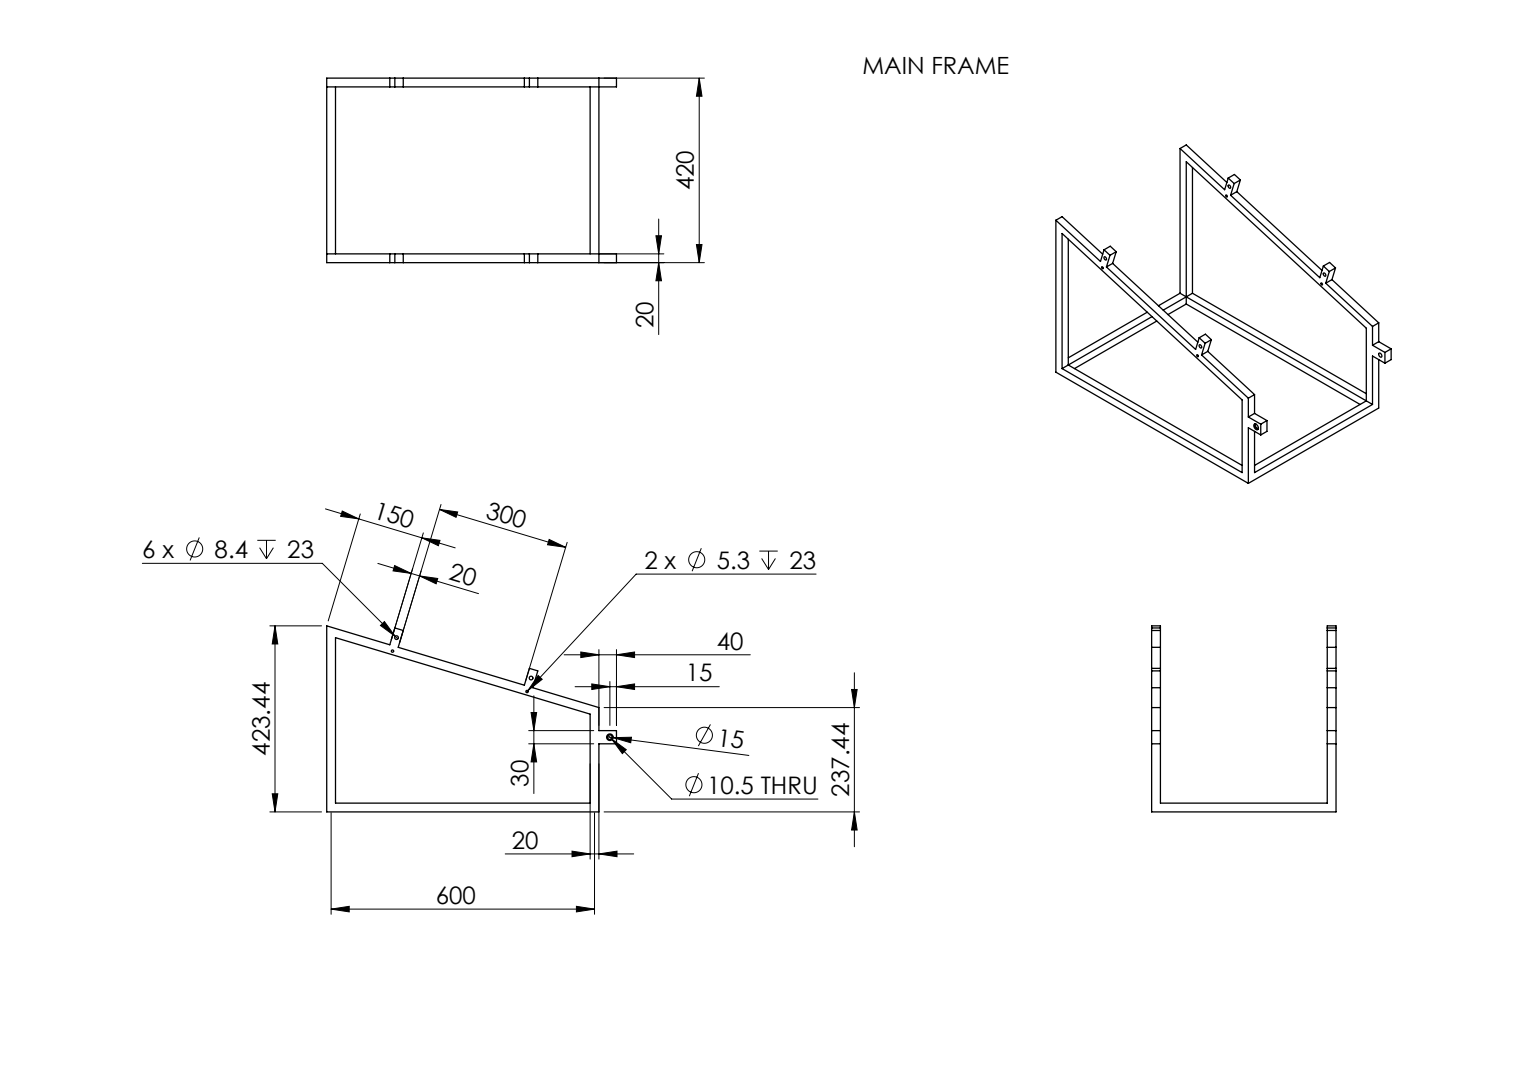
ISO-10303-21;
HEADER;
FILE_DESCRIPTION (('STEP AP214'),
    '1' );
FILE_NAME ('main frame.step',
    '2026-10-27T17:01:19',
    ( '' ),
    ( '' ),
    'SwSTEP 2.0',
    'SolidWorks 2026',
    '' );
FILE_SCHEMA (( 'AUTOMOTIVE_DESIGN' ));
ENDSEC;

DATA;
#2=DIRECTION ( 'NONE',  ( 1.000000000000000000, 0.000000000000000000, 0.000000000000000000 ) ) ;
#7=EDGE_CURVE ( 'NONE', #11993, #2660, #12348, .T. ) ;
#12=ORIENTED_EDGE ( 'NONE', *, *, #9612, .F. ) ;
#21=CARTESIAN_POINT ( 'NONE',  ( 148.9991633467111569, 386.6211705227183870, -190.0000000000000000 ) ) ;
#26=DIRECTION ( 'NONE',  ( 0.000000000000000000, 0.000000000000000000, 1.000000000000000000 ) ) ;
#34=EDGE_CURVE ( 'NONE', #1936, #10044, #4903, .T. ) ;
#41=CARTESIAN_POINT ( 'NONE',  ( 164.3243839102495656, 402.9042173714779551, -210.0000000000000000 ) ) ;
#50=EDGE_LOOP ( 'NONE', ( #5774, #9979, #12011, #287 ) ) ;
#54=VERTEX_POINT ( 'NONE', #6074 ) ;
#72=VERTEX_POINT ( 'NONE', #2614 ) ;
#74=EDGE_LOOP ( 'NONE', ( #5773, #12707 ) ) ;
#76=CARTESIAN_POINT ( 'NONE',  ( 451.6722694765949768, 316.6998517015743460, -210.0000000000000000 ) ) ;
#79=CARTESIAN_POINT ( 'NONE',  ( 650.0000000000000000, 175.0000000000000568, 190.0000000000000000 ) ) ;
#80=CARTESIAN_POINT ( 'NONE',  ( 459.7035746174795463, 294.6698471414878782, 210.0000000000000000 ) ) ;
#82=DIRECTION ( 'NONE',  ( 1.000000000000000000, 0.000000000000000000, 0.000000000000000000 ) ) ;
#84=ORIENTED_EDGE ( 'NONE', *, *, #4575, .F. ) ;
#85=CARTESIAN_POINT ( 'NONE',  ( 642.5000000000001137, 160.0000000000000284, -207.0000000000000000 ) ) ;
#90=DIRECTION ( 'NONE',  ( 1.000000000000000000, 0.000000000000000000, 0.000000000000000000 ) ) ;
#103=CARTESIAN_POINT ( 'NONE',  ( 642.4999005938085475, 159.0059381730093548, -210.0000000000000284 ) ) ;
#104=CARTESIAN_POINT ( 'NONE',  ( 642.5000000000001137, 160.0000000000000284, 210.0000119999999981 ) ) ;
#105=LINE ( 'NONE', #11206, #8037 ) ;
#116=CARTESIAN_POINT ( 'NONE',  ( 145.1678582058265476, 408.6511750828048548, -190.0000000000000000 ) ) ;
#130=EDGE_CURVE ( 'NONE', #2847, #2989, #365, .T. ) ;
#132=CARTESIAN_POINT ( 'NONE',  ( 610.0000000000000000, 0.000000000000000000, -210.0000000000000000 ) ) ;
#134=CARTESIAN_POINT ( 'NONE',  ( 650.0000000000000000, 0.000000000000000000, 0.000000000000000000 ) ) ;
#137=CARTESIAN_POINT ( 'NONE',  ( 641.5533979126569193, 156.2228576472182624, 210.0000119999999981 ) ) ;
#140=CARTESIAN_POINT ( 'NONE',  ( 9.498873539028489220E-16, -10.00000000000000000, 210.0000000000000000 ) ) ;
#144=VECTOR ( 'NONE', #10565, 1000.000000000000000 ) ;
#145=VERTEX_POINT ( 'NONE', #14118 ) ;
#153=EDGE_LOOP ( 'NONE', ( #10187, #6954 ) ) ;
#165=CARTESIAN_POINT ( 'NONE',  ( 459.3348797583642522, 272.6398425814014104, -210.0000000000000000 ) ) ;
#176=VECTOR ( 'NONE', #3313, 1000.000000000000000 ) ;
#180=ORIENTED_EDGE ( 'NONE', *, *, #12151, .F. ) ;
#187=ORIENTED_EDGE ( 'NONE', *, *, #791, .F. ) ;
#197=VERTEX_POINT ( 'NONE', #7549 ) ;
#202=VECTOR ( 'NONE', #5695, 1000.000000000000000 ) ;
#205=LINE ( 'NONE', #12625, #7486 ) ;
#210=DIRECTION ( 'NONE',  ( 0.000000000000000000, 0.000000000000000000, 1.000000000000000000 ) ) ;
#213=DIRECTION ( 'NONE',  ( 0.000000000000000000, -0.000000000000000000, -1.000000000000000000 ) ) ;
#214=VERTEX_POINT ( 'NONE', #14200 ) ;
#216=CARTESIAN_POINT ( 'NONE',  ( 640.9975013179864618, 155.3908996001881064, 210.0000119999999981 ) ) ;
#217=CARTESIAN_POINT ( 'NONE',  ( 145.1678582058265192, 408.6511750828049117, 210.0000000000000000 ) ) ;
#235=AXIS2_PLACEMENT_3D ( 'NONE', #506, #13872, #10410 ) ;
#236=DIRECTION ( 'NONE',  ( 0.000000000000000000, 0.000000000000000000, 1.000000000000000000 ) ) ;
#244=DIRECTION ( 'NONE',  ( 0.9578262852211513190, -0.2873478855663453846, 0.000000000000000000 ) ) ;
#254=CARTESIAN_POINT ( 'NONE',  ( 10.00000000000000000, 0.000000000000000000, 210.0000000000000000 ) ) ;
#257=ORIENTED_EDGE ( 'NONE', *, *, #4905, .T. ) ;
#258=CARTESIAN_POINT ( 'NONE',  ( 10.00000000000000000, 386.5596934910894902, -190.0000000000000000 ) ) ;
#261=LINE ( 'NONE', #1530, #10839 ) ;
#262=DIRECTION ( 'NONE',  ( -0.000000000000000000, -0.000000000000000000, -1.000000000000000000 ) ) ;
#263=VECTOR ( 'NONE', #2526, 1000.000000000000000 ) ;
#265=CARTESIAN_POINT ( 'NONE',  ( 459.7035746174795463, 294.6698471414878782, -210.0000000000000000 ) ) ;
#281=EDGE_CURVE ( 'NONE', #5961, #525, #3049, .T. ) ;
#283=CARTESIAN_POINT ( 'NONE',  ( 112.9652219749295341, 376.5507399164317803, -190.0000000000000000 ) ) ;
#285=VECTOR ( 'NONE', #13609, 1000.000000000000000 ) ;
#287=ORIENTED_EDGE ( 'NONE', *, *, #8174, .T. ) ;
#291=LINE ( 'NONE', #8346, #11794 ) ;
#292=ORIENTED_EDGE ( 'NONE', *, *, #6303, .T. ) ;
#300=CARTESIAN_POINT ( 'NONE',  ( 650.0000000000000000, 175.0000000000000568, 210.0000000000000000 ) ) ;
#311=EDGE_CURVE ( 'NONE', #1794, #10356, #7010, .T. ) ;
#313=LINE ( 'NONE', #2471, #1913 ) ;
#320=CARTESIAN_POINT ( 'NONE',  ( 440.1783540539412343, 278.3868002927283101, -190.0000000000000000 ) ) ;
#322=EDGE_CURVE ( 'NONE', #11174, #11494, #10043, .T. ) ;
#324=VECTOR ( 'NONE', #11210, 1000.000000000000000 ) ;
#326=ORIENTED_EDGE ( 'NONE', *, *, #6236, .F. ) ;
#336=CARTESIAN_POINT ( 'NONE',  ( 145.1678582058265192, 408.6511750828049117, 210.0000000000000000 ) ) ;
#337=ORIENTED_EDGE ( 'NONE', *, *, #5739, .T. ) ;
#338=FACE_OUTER_BOUND ( 'NONE', #7888, .T. ) ;
#343=ORIENTED_EDGE ( 'NONE', *, *, #2161, .T. ) ;
#347=EDGE_CURVE ( 'NONE', #8605, #12947, #205, .T. ) ;
#352=VERTEX_POINT ( 'NONE', #14549 ) ;
#359=EDGE_LOOP ( 'NONE', ( #3831, #5633, #326, #12007 ) ) ;
#363=ORIENTED_EDGE ( 'NONE', *, *, #918, .F. ) ;
#365=LINE ( 'NONE', #2825, #10917 ) ;
#384=FACE_OUTER_BOUND ( 'NONE', #5110, .T. ) ;
#385=ORIENTED_EDGE ( 'NONE', *, *, #3968, .F. ) ;
#386=CARTESIAN_POINT ( 'NONE',  ( 10.00000000000000000, 386.5596934910894902, 210.0000000000000000 ) ) ;
#387=LINE ( 'NONE', #4789, #930 ) ;
#393=ORIENTED_EDGE ( 'NONE', *, *, #10167, .F. ) ;
#396=ORIENTED_EDGE ( 'NONE', *, *, #10216, .T. ) ;
#397=EDGE_CURVE ( 'NONE', #6493, #1729, #8054, .T. ) ;
#398=CIRCLE ( 'NONE', #12374, 4.200000000000009059 ) ;
#413=DIRECTION ( 'NONE',  ( -0.9578262852211513190, 0.2873478855663453846, 0.000000000000000000 ) ) ;
#414=ORIENTED_EDGE ( 'NONE', *, *, #14037, .F. ) ;
#417=ORIENTED_EDGE ( 'NONE', *, *, #9564, .F. ) ;
#432=AXIS2_PLACEMENT_3D ( 'NONE', #1047, #4454, #8952 ) ;
#437=CARTESIAN_POINT ( 'NONE',  ( 610.0000000000000000, 10.00000000000005507, -190.0000000000000000 ) ) ;
#441=CARTESIAN_POINT ( 'NONE',  ( 650.0000000000000000, 175.0000000000000568, -210.0000000000000000 ) ) ;
#444=CARTESIAN_POINT ( 'NONE',  ( 642.3047950750122936, 158.0368908673054023, 210.0000119999999981 ) ) ;
#459=LINE ( 'NONE', #6230, #3858 ) ;
#463=DIRECTION ( 'NONE',  ( 0.000000000000000000, 0.000000000000000000, -1.000000000000000000 ) ) ;
#466=AXIS2_PLACEMENT_3D ( 'NONE', #4153, #9690, #6360 ) ;
#472=EDGE_CURVE ( 'NONE', #11723, #11023, #398, .T. ) ;
#473=CARTESIAN_POINT ( 'NONE',  ( 459.7035746174796031, 294.6698471414878782, 210.0000000000000000 ) ) ;
#476=ORIENTED_EDGE ( 'NONE', *, *, #1979, .F. ) ;
#480=DIRECTION ( 'NONE',  ( -0.000000000000000000, -0.000000000000000000, -1.000000000000000000 ) ) ;
#484=VECTOR ( 'NONE', #9358, 1000.000000000000000 ) ;
#489=VECTOR ( 'NONE', #7910, 1000.000000000000114 ) ;
#493=EDGE_CURVE ( 'NONE', #6798, #4861, #9598, .T. ) ;
#498=EDGE_CURVE ( 'NONE', #10448, #9080, #1487, .T. ) ;
#499=CARTESIAN_POINT ( 'NONE',  ( 635.0000000000000000, 160.0000000000000284, -210.0000000000000000 ) ) ;
#503=VERTEX_POINT ( 'NONE', #14036 ) ;
#506=CARTESIAN_POINT ( 'NONE',  ( 455.5035746174796714, 294.6698471414878782, -210.0000000000000000 ) ) ;
#517=EDGE_LOOP ( 'NONE', ( #8251, #6381, #5116, #1964 ) ) ;
#525=VERTEX_POINT ( 'NONE', #9313 ) ;
#528=DIRECTION ( 'NONE',  ( -1.000000000000000000, 0.000000000000000000, 0.000000000000000000 ) ) ;
#529=VECTOR ( 'NONE', #13044, 1000.000000000000000 ) ;
#534=CYLINDRICAL_SURFACE ( 'NONE', #9490, 4.199999999999926459 ) ;
#536=CARTESIAN_POINT ( 'NONE',  ( 650.0000000000000000, 145.0000000000000568, -210.0000000000000000 ) ) ;
#542=VERTEX_POINT ( 'NONE', #1550 ) ;
#550=DIRECTION ( 'NONE',  ( 0.9578262852211513190, -0.2873478855663453846, 0.000000000000000000 ) ) ;
#562=FACE_BOUND ( 'NONE', #4810, .T. ) ;
#565=ORIENTED_EDGE ( 'NONE', *, *, #4113, .T. ) ;
#577=CARTESIAN_POINT ( 'NONE',  ( 590.0000000000000000, -9.999999999999941380, -190.0000000000000000 ) ) ;
#586=ORIENTED_EDGE ( 'NONE', *, *, #12930, .F. ) ;
#589=CARTESIAN_POINT ( 'NONE',  ( 610.0000000000000000, 0.000000000000000000, 210.0000000000000000 ) ) ;
#594=ADVANCED_FACE ( 'NONE', ( #8569 ), #6567, .F. ) ;
#606=CARTESIAN_POINT ( 'NONE',  ( 451.3035746174797396, 294.6698471414878782, 210.0000000000000000 ) ) ;
#608=DIRECTION ( 'NONE',  ( 0.000000000000000000, 0.000000000000000000, -1.000000000000000000 ) ) ;
#613=CARTESIAN_POINT ( 'NONE',  ( 639.6091003998118367, 165.9975013179864334, 210.0000119999999981 ) ) ;
#619=PLANE ( 'NONE',  #5173 ) ;
#620=ORIENTED_EDGE ( 'NONE', *, *, #10389, .T. ) ;
#624=DIRECTION ( 'NONE',  ( -0.000000000000000000, -0.000000000000000000, -1.000000000000000000 ) ) ;
#634=( NAMED_UNIT ( * ) SI_UNIT ( $, .STERADIAN. ) SOLID_ANGLE_UNIT ( ) );
#646=CARTESIAN_POINT ( 'NONE',  ( 639.6004632909515522, 166.0062790084377013, -210.0000000000000000 ) ) ;
#650=ORIENTED_EDGE ( 'NONE', *, *, #6792, .F. ) ;
#656=CARTESIAN_POINT ( 'NONE',  ( 112.9652219749295341, 376.5507399164317803, 210.0000000000000000 ) ) ;
#657=ORIENTED_EDGE ( 'NONE', *, *, #4005, .F. ) ;
#674=PLANE ( 'NONE',  #14348 ) ;
#675=EDGE_LOOP ( 'NONE', ( #11557, #8430, #2756, #7355 ) ) ;
#685=DIRECTION ( 'NONE',  ( 0.000000000000000000, 1.000000000000000000, 0.000000000000000000 ) ) ;
#691=CARTESIAN_POINT ( 'NONE',  ( 631.2228576472183477, 166.5533979126570330, 210.0000119999999981 ) ) ;
#703=CIRCLE ( 'NONE', #8021, 4.199999999999981526 ) ;
#713=CARTESIAN_POINT ( 'NONE',  ( 142.4540310085880606, 355.9707293956415697, -210.0000000000000000 ) ) ;
#722=ORIENTED_EDGE ( 'NONE', *, *, #12878, .F. ) ;
#725=DIRECTION ( 'NONE',  ( -1.000000000000000000, 0.000000000000000000, 0.000000000000000000 ) ) ;
#735=DIRECTION ( 'NONE',  ( 1.000000000000000000, 0.000000000000000000, 0.000000000000000000 ) ) ;
#739=VERTEX_POINT ( 'NONE', #10988 ) ;
#750=ORIENTED_EDGE ( 'NONE', *, *, #10896, .T. ) ;
#757=CARTESIAN_POINT ( 'NONE',  ( 640.2500000000000000, 160.0000000000000284, -190.0000000000000000 ) ) ;
#770=ORIENTED_EDGE ( 'NONE', *, *, #10512, .T. ) ;
#776=VECTOR ( 'NONE', #6967, 1000.000000000000000 ) ;
#779=CYLINDRICAL_SURFACE ( 'NONE', #2321, 7.500000000000062172 ) ;
#780=ORIENTED_EDGE ( 'NONE', *, *, #4466, .T. ) ;
#781=FACE_OUTER_BOUND ( 'NONE', #3795, .T. ) ;
#791=EDGE_CURVE ( 'NONE', #6358, #5212, #2203, .T. ) ;
#793=VERTEX_POINT ( 'NONE', #5751 ) ;
#799=DIRECTION ( 'NONE',  ( -1.000000000000000000, 0.000000000000000000, 0.000000000000000000 ) ) ;
#800=CARTESIAN_POINT ( 'NONE',  ( 446.3084422793565409, 264.0194060144110608, -210.0000000000000000 ) ) ;
#804=CARTESIAN_POINT ( 'NONE',  ( 451.6722694765949768, 316.6998517015743460, -190.0000000000000000 ) ) ;
#813=PLANE ( 'NONE',  #12711 ) ;
#819=ADVANCED_FACE ( 'NONE', ( #11141 ), #13509, .T. ) ;
#830=ORIENTED_EDGE ( 'NONE', *, *, #10724, .T. ) ;
#842=ORIENTED_EDGE ( 'NONE', *, *, #9433, .T. ) ;
#848=LINE ( 'NONE', #5367, #4476 ) ;
#850=CARTESIAN_POINT ( 'NONE',  ( 627.5000000000000000, 160.0000000000000284, -210.0000119999999981 ) ) ;
#851=( LENGTH_UNIT ( ) NAMED_UNIT ( * ) SI_UNIT ( .MILLI., .METRE. ) );
#854=LINE ( 'NONE', #14242, #1628 ) ;
#857=ORIENTED_EDGE ( 'NONE', *, *, #6432, .F. ) ;
#871=ADVANCED_FACE ( 'NONE', ( #11787 ), #7070, .F. ) ;
#881=FACE_OUTER_BOUND ( 'NONE', #6176, .T. ) ;
#885=VECTOR ( 'NONE', #12868, 1000.000000000000000 ) ;
#902=VERTEX_POINT ( 'NONE', #5973 ) ;
#915=LINE ( 'NONE', #5298, #3326 ) ;
#918=EDGE_CURVE ( 'NONE', #12905, #9301, #11493, .T. ) ;
#919=VECTOR ( 'NONE', #3316, 1000.000000000000000 ) ;
#922=DIRECTION ( 'NONE',  ( -0.2873478855663453846, -0.9578262852211513190, -0.000000000000000000 ) ) ;
#928=ORIENTED_EDGE ( 'NONE', *, *, #12930, .T. ) ;
#929=AXIS2_PLACEMENT_3D ( 'NONE', #5591, #6707, #6495 ) ;
#930=VECTOR ( 'NONE', #8229, 1000.000000000000000 ) ;
#932=ORIENTED_EDGE ( 'NONE', *, *, #311, .T. ) ;
#937=CARTESIAN_POINT ( 'NONE',  ( 153.1991633467111456, 386.6211705227183870, 210.0000000000000000 ) ) ;
#938=CARTESIAN_POINT ( 'NONE',  ( 628.9937209914679670, 164.6004632908573342, -210.0000000000000000 ) ) ;
#947=VECTOR ( 'NONE', #14401, 1000.000000000000227 ) ;
#959=CARTESIAN_POINT ( 'NONE',  ( 590.0000000000000000, 10.00000000000005507, 210.0000000000000000 ) ) ;
#970=EDGE_CURVE ( 'NONE', #9080, #2989, #1606, .T. ) ;
#974=LINE ( 'NONE', #12475, #9641 ) ;
#976=CIRCLE ( 'NONE', #8526, 2.649999999999985700 ) ;
#980=DIRECTION ( 'NONE',  ( 0.000000000000000000, -1.000000000000000000, 0.000000000000000000 ) ) ;
#988=AXIS2_PLACEMENT_3D ( 'NONE', #13184, #5359, #12203 ) ;
#990=FACE_OUTER_BOUND ( 'NONE', #11899, .T. ) ;
#994=ORIENTED_EDGE ( 'NONE', *, *, #11063, .T. ) ;
#996=CARTESIAN_POINT ( 'NONE',  ( 10.00000000000000000, -10.00000000000000000, 190.0000000000000000 ) ) ;
#1000=EDGE_CURVE ( 'NONE', #10070, #5539, #3911, .T. ) ;
#1003=CYLINDRICAL_SURFACE ( 'NONE', #11112, 7.500000000000062172 ) ;
#1009=DIRECTION ( 'NONE',  ( 1.000000000000000000, 0.000000000000000000, -0.000000000000000000 ) ) ;
#1017=CARTESIAN_POINT ( 'NONE',  ( 627.5000000000000000, 160.9948216655610622, -210.0000000000000284 ) ) ;
#1025=LINE ( 'NONE', #1991, #8652 ) ;
#1027=FACE_OUTER_BOUND ( 'NONE', #1102, .T. ) ;
#1031=ORIENTED_EDGE ( 'NONE', *, *, #1242, .F. ) ;
#1037=EDGE_LOOP ( 'NONE', ( #8781, #13398, #8659, #1616 ) ) ;
#1038=CARTESIAN_POINT ( 'NONE',  ( 443.6584422793565636, 264.0194060144110608, -190.0000000000000000 ) ) ;
#1047=CARTESIAN_POINT ( 'NONE',  ( 455.5035746174796714, 294.6698471414878782, -190.0000000000000000 ) ) ;
#1054=DIRECTION ( 'NONE',  ( -0.000000000000000000, -0.000000000000000000, 1.000000000000000000 ) ) ;
#1055=DIRECTION ( 'NONE',  ( -0.9578262852211517631, 0.2873478855663438858, 0.000000000000000000 ) ) ;
#1062=ORIENTED_EDGE ( 'NONE', *, *, #347, .F. ) ;
#1064=CARTESIAN_POINT ( 'NONE',  ( 451.6722694765949768, 316.6998517015743460, -210.0000000000000000 ) ) ;
#1066=ADVANCED_FACE ( 'NONE', ( #9586 ), #6607, .T. ) ;
#1073=CARTESIAN_POINT ( 'NONE',  ( -10.00000000000000000, 0.000000000000000000, -190.0000000000000000 ) ) ;
#1076=( LENGTH_UNIT ( ) NAMED_UNIT ( * ) SI_UNIT ( .MILLI., .METRE. ) );
#1084=FACE_OUTER_BOUND ( 'NONE', #6931, .T. ) ;
#1085=CARTESIAN_POINT ( 'NONE',  ( 630.3996772907336208, 166.0061384269410212, -210.0000000000000284 ) ) ;
#1102=EDGE_LOOP ( 'NONE', ( #5350, #8471, #4315, #12302 ) ) ;
#1104=ORIENTED_EDGE ( 'NONE', *, *, #7956, .T. ) ;
#1111=ORIENTED_EDGE ( 'NONE', *, *, #1647, .T. ) ;
#1123=CARTESIAN_POINT ( 'NONE',  ( 10.00000000000000000, 386.5596934910894902, 210.0000000000000000 ) ) ;
#1124=EDGE_CURVE ( 'NONE', #10210, #9473, #7995, .T. ) ;
#1126=LINE ( 'NONE', #5639, #9616 ) ;
#1129=ORIENTED_EDGE ( 'NONE', *, *, #11458, .T. ) ;
#1138=VERTEX_POINT ( 'NONE', #12577 ) ;
#1145=CARTESIAN_POINT ( 'NONE',  ( 635.0000000000000000, 160.0000000000000284, 190.0000000000000284 ) ) ;
#1146=EDGE_CURVE ( 'NONE', #503, #13396, #5852, .T. ) ;
#1149=ORIENTED_EDGE ( 'NONE', *, *, #11070, .T. ) ;
#1152=CARTESIAN_POINT ( 'NONE',  ( 459.3348797583643091, 272.6398425814014104, -190.0000000000000000 ) ) ;
#1156=CIRCLE ( 'NONE', #13898, 4.199999999999981526 ) ;
#1158=DIRECTION ( 'NONE',  ( -0.000000000000000000, -0.000000000000000000, -1.000000000000000000 ) ) ;
#1181=LINE ( 'NONE', #959, #202 ) ;
#1182=CIRCLE ( 'NONE', #4025, 2.649999999999985700 ) ;
#1183=CARTESIAN_POINT ( 'NONE',  ( 650.0000000000000000, 145.0000000000000568, -190.0000000000000000 ) ) ;
#1185=CARTESIAN_POINT ( 'NONE',  ( 451.6722694765949768, 316.6998517015743460, 190.0000000000000000 ) ) ;
#1189=DIRECTION ( 'NONE',  ( 0.000000000000000000, 1.000000000000000000, 0.000000000000000000 ) ) ;
#1194=EDGE_LOOP ( 'NONE', ( #13478, #6976 ) ) ;
#1195=ORIENTED_EDGE ( 'NONE', *, *, #13922, .T. ) ;
#1198=VECTOR ( 'NONE', #12811, 1000.000000000000114 ) ;
#1205=ORIENTED_EDGE ( 'NONE', *, *, #4135, .F. ) ;
#1208=CIRCLE ( 'NONE', #13243, 7.500000000000062172 ) ;
#1211=CARTESIAN_POINT ( 'NONE',  ( 148.9991633467111569, 386.6211705227183870, 210.0000000000000000 ) ) ;
#1227=DIRECTION ( 'NONE',  ( -0.2873478855663453846, -0.9578262852211513190, -0.000000000000000000 ) ) ;
#1229=EDGE_LOOP ( 'NONE', ( #830, #13146 ) ) ;
#1242=EDGE_CURVE ( 'NONE', #72, #3152, #10578, .T. ) ;
#1244=CARTESIAN_POINT ( 'NONE',  ( 638.7885571598276329, 153.4512226587835642, -210.0000000000000000 ) ) ;
#1246=DIRECTION ( 'NONE',  ( 1.000000000000000000, 0.000000000000000000, 0.000000000000000000 ) ) ;
#1249=CARTESIAN_POINT ( 'NONE',  ( 112.9652219749295341, 376.5507399164317803, 210.0000000000000000 ) ) ;
#1251=DIRECTION ( 'NONE',  ( -0.9578262852211513190, 0.2873478855663453846, 0.000000000000000000 ) ) ;
#1260=VECTOR ( 'NONE', #3658, 1000.000000000000000 ) ;
#1262=ORIENTED_EDGE ( 'NONE', *, *, #8034, .T. ) ;
#1265=FACE_OUTER_BOUND ( 'NONE', #4449, .T. ) ;
#1267=LINE ( 'NONE', #577, #4034 ) ;
#1272=DIRECTION ( 'NONE',  ( 1.387778780781446464E-15, -2.775557561562892929E-15, 1.000000000000000000 ) ) ;
#1277=CARTESIAN_POINT ( 'NONE',  ( 630.3908996001882770, 154.0024986820136803, 210.0000119999999981 ) ) ;
#1289=ORIENTED_EDGE ( 'NONE', *, *, #8696, .F. ) ;
#1290=DIRECTION ( 'NONE',  ( -0.000000000000000000, -0.000000000000000000, 1.000000000000000000 ) ) ;
#1294=DIRECTION ( 'NONE',  ( -1.000000000000000000, -9.498873539028489960E-17, -0.000000000000000000 ) ) ;
#1297=PLANE ( 'NONE',  #3818 ) ;
#1299=PLANE ( 'NONE',  #13009 ) ;
#1306=FACE_OUTER_BOUND ( 'NONE', #4104, .T. ) ;
#1308=ORIENTED_EDGE ( 'NONE', *, *, #9612, .T. ) ;
#1313=DIRECTION ( 'NONE',  ( 0.000000000000000000, 0.000000000000000000, 1.000000000000000000 ) ) ;
#1319=VERTEX_POINT ( 'NONE', #10502 ) ;
#1326=EDGE_CURVE ( 'NONE', #12898, #12523, #9621, .T. ) ;
#1335=EDGE_CURVE ( 'NONE', #8820, #739, #4018, .T. ) ;
#1342=ORIENTED_EDGE ( 'NONE', *, *, #9115, .F. ) ;
#1356=PLANE ( 'NONE',  #5436 ) ;
#1358=EDGE_LOOP ( 'NONE', ( #5343, #14402, #10147, #3262 ) ) ;
#1378=VECTOR ( 'NONE', #1272, 1000.000000000000000 ) ;
#1379=CARTESIAN_POINT ( 'NONE',  ( 642.3095993250867650, 158.0482295922596450, -210.0000000000000000 ) ) ;
#1385=CARTESIAN_POINT ( 'NONE',  ( 459.3348797583642522, 272.6398425814014104, -210.0000000000000000 ) ) ;
#1394=ORIENTED_EDGE ( 'NONE', *, *, #5211, .F. ) ;
#1398=ORIENTED_EDGE ( 'NONE', *, *, #3960, .T. ) ;
#1402=DIRECTION ( 'NONE',  ( -0.000000000000000000, -0.000000000000000000, -1.000000000000000000 ) ) ;
#1407=DIRECTION ( 'NONE',  ( -0.000000000000000000, -0.000000000000000000, 1.000000000000000000 ) ) ;
#1414=VECTOR ( 'NONE', #13789, 1000.000000000000114 ) ;
#1416=AXIS2_PLACEMENT_3D ( 'NONE', #12274, #4328, #9037 ) ;
#1425=EDGE_CURVE ( 'NONE', #10194, #525, #4233, .T. ) ;
#1428=EDGE_CURVE ( 'NONE', #12947, #2635, #10045, .T. ) ;
#1437=AXIS2_PLACEMENT_3D ( 'NONE', #800, #13135, #14530 ) ;
#1438=ORIENTED_EDGE ( 'NONE', *, *, #12056, .T. ) ;
#1444=VECTOR ( 'NONE', #262, 1000.000000000000000 ) ;
#1447=AXIS2_PLACEMENT_3D ( 'NONE', #13346, #3239, #1833 ) ;
#1451=DIRECTION ( 'NONE',  ( 1.000000000000000000, 0.000000000000000000, 0.000000000000000000 ) ) ;
#1458=DIRECTION ( 'NONE',  ( 1.000000000000000000, -0.000000000000000000, -0.000000000000000000 ) ) ;
#1461=CIRCLE ( 'NONE', #5465, 4.199999999999981526 ) ;
#1477=DIRECTION ( 'NONE',  ( 0.000000000000000000, 0.000000000000000000, 1.000000000000000000 ) ) ;
#1484=ADVANCED_FACE ( 'NONE', ( #1861 ), #6588, .F. ) ;
#1487=LINE ( 'NONE', #1623, #5551 ) ;
#1496=CARTESIAN_POINT ( 'NONE',  ( 451.3035746174797396, 294.6698471414878782, -210.0000000000000000 ) ) ;
#1499=EDGE_CURVE ( 'NONE', #902, #7765, #3348, .T. ) ;
#1507=CARTESIAN_POINT ( 'NONE',  ( 137.1540310085880776, 355.9707293956415697, -210.0000000000000000 ) ) ;
#1520=LINE ( 'NONE', #386, #8999 ) ;
#1527=DIRECTION ( 'NONE',  ( 1.000000000000000000, 0.000000000000000000, -0.000000000000000000 ) ) ;
#1530=CARTESIAN_POINT ( 'NONE',  ( 650.0000000000000000, 175.0000000000000568, -210.0000000000000000 ) ) ;
#1531=CARTESIAN_POINT ( 'NONE',  ( 455.5035746174796714, 294.6698471414878782, 190.0000000000000000 ) ) ;
#1538=VERTEX_POINT ( 'NONE', #11162 ) ;
#1544=VERTEX_POINT ( 'NONE', #1038 ) ;
#1550=CARTESIAN_POINT ( 'NONE',  ( 152.8304684875957378, 364.5911659626319192, 190.0000000000000000 ) ) ;
#1553=FACE_BOUND ( 'NONE', #8777, .T. ) ;
#1559=DIRECTION ( 'NONE',  ( -1.000000000000000000, -0.000000000000000000, -0.000000000000000000 ) ) ;
#1561=CARTESIAN_POINT ( 'NONE',  ( 610.0000000000000000, 227.4403065089105951, -210.0000000000000000 ) ) ;
#1566=LINE ( 'NONE', #9179, #4728 ) ;
#1591=LINE ( 'NONE', #10682, #4472 ) ;
#1606=LINE ( 'NONE', #4809, #9482 ) ;
#1610=EDGE_LOOP ( 'NONE', ( #4110, #12927, #11663, #6845 ) ) ;
#1616=ORIENTED_EDGE ( 'NONE', *, *, #10512, .F. ) ;
#1623=CARTESIAN_POINT ( 'NONE',  ( 590.0000000000000000, 212.5596934910894333, -210.0000000000000000 ) ) ;
#1628=VECTOR ( 'NONE', #7598, 1000.000000000000114 ) ;
#1638=PLANE ( 'NONE',  #4224 ) ;
#1647=EDGE_CURVE ( 'NONE', #11118, #10957, #11227, .T. ) ;
#1658=AXIS2_PLACEMENT_3D ( 'NONE', #6165, #10667, #463 ) ;
#1665=ORIENTED_EDGE ( 'NONE', *, *, #8262, .F. ) ;
#1673=ORIENTED_EDGE ( 'NONE', *, *, #4100, .F. ) ;
#1679=CIRCLE ( 'NONE', #9928, 2.649999999999985700 ) ;
#1682=DIRECTION ( 'NONE',  ( 0.000000000000000000, 0.000000000000000000, 1.000000000000000000 ) ) ;
#1685=ORIENTED_EDGE ( 'NONE', *, *, #1425, .T. ) ;
#1690=CARTESIAN_POINT ( 'NONE',  ( 440.1783540539412343, 278.3868002927283101, 210.0000000000000000 ) ) ;
#1703=CARTESIAN_POINT ( 'NONE',  ( 112.9652219749295341, 376.5507399164317803, 210.0000000000000000 ) ) ;
#1707=CARTESIAN_POINT ( 'NONE',  ( 148.9991633467111569, 386.6211705227183870, 210.0000000000000000 ) ) ;
#1729=VERTEX_POINT ( 'NONE', #1770 ) ;
#1732=ORIENTED_EDGE ( 'NONE', *, *, #498, .F. ) ;
#1741=CARTESIAN_POINT ( 'NONE',  ( 148.9991633467111569, 386.6211705227183870, -210.0000000000000000 ) ) ;
#1746=ORIENTED_EDGE ( 'NONE', *, *, #3611, .F. ) ;
#1750=CARTESIAN_POINT ( 'NONE',  ( 627.5000000000000000, 160.0000000000000284, 207.0000000000000000 ) ) ;
#1751=ORIENTED_EDGE ( 'NONE', *, *, #5498, .F. ) ;
#1752=DIRECTION ( 'NONE',  ( 1.000000000000000000, 9.498873539028489960E-17, 0.000000000000000000 ) ) ;
#1763=CARTESIAN_POINT ( 'NONE',  ( 642.5000994061915662, 160.9940618269907020, -209.9999999999999716 ) ) ;
#1770=CARTESIAN_POINT ( 'NONE',  ( 451.6722694765949768, 316.6998517015743460, 190.0000000000000000 ) ) ;
#1775=EDGE_LOOP ( 'NONE', ( #12688, #11502, #5375, #9233 ) ) ;
#1776=CYLINDRICAL_SURFACE ( 'NONE', #10557, 4.199999999999981526 ) ;
#1784=EDGE_CURVE ( 'NONE', #3368, #1845, #5988, .T. ) ;
#1794=VERTEX_POINT ( 'NONE', #437 ) ;
#1798=CARTESIAN_POINT ( 'NONE',  ( 635.0000000000000000, 160.0000000000000284, -207.0000000000000000 ) ) ;
#1804=DIRECTION ( 'NONE',  ( -1.000000000000000000, 0.000000000000000000, 0.000000000000000000 ) ) ;
#1813=DIRECTION ( 'NONE',  ( 0.000000000000000000, 1.000000000000000000, 0.000000000000000000 ) ) ;
#1818=AXIS2_PLACEMENT_3D ( 'NONE', #1741, #480, #11630 ) ;
#1832=LINE ( 'NONE', #2888, #9216 ) ;
#1833=DIRECTION ( 'NONE',  ( 1.000000000000000000, 0.000000000000000000, 0.000000000000000000 ) ) ;
#1836=VERTEX_POINT ( 'NONE', #9467 ) ;
#1841=DIRECTION ( 'NONE',  ( 0.000000000000000000, 0.000000000000000000, 1.000000000000000000 ) ) ;
#1845=VERTEX_POINT ( 'NONE', #6213 ) ;
#1855=CARTESIAN_POINT ( 'NONE',  ( 610.0000000000000000, 0.000000000000000000, 190.0000000000000000 ) ) ;
#1861=FACE_OUTER_BOUND ( 'NONE', #4687, .T. ) ;
#1871=CARTESIAN_POINT ( 'NONE',  ( 590.0000000000000000, 212.5596934910894333, -190.0000000000000000 ) ) ;
#1872=ADVANCED_FACE ( 'NONE', ( #4292 ), #6434, .T. ) ;
#1873=SHAPE_REPRESENTATION ( 'main frame', ( #9440 ), #7553 ) ;
#1877=AXIS2_PLACEMENT_3D ( 'NONE', #12827, #1682, #13942 ) ;
#1884=DIRECTION ( 'NONE',  ( 0.000000000000000000, 0.000000000000000000, -1.000000000000000000 ) ) ;
#1889=FACE_OUTER_BOUND ( 'NONE', #13103, .T. ) ;
#1895=VECTOR ( 'NONE', #8715, 1000.000000000000114 ) ;
#1896=CARTESIAN_POINT ( 'NONE',  ( 629.7500000000000000, 160.0000000000000284, -210.0000000000000000 ) ) ;
#1903=DIRECTION ( 'NONE',  ( 0.000000000000000000, 0.000000000000000000, 1.000000000000000000 ) ) ;
#1913=VECTOR ( 'NONE', #90, 1000.000000000000000 ) ;
#1915=DIRECTION ( 'NONE',  ( -0.000000000000000000, -0.000000000000000000, 1.000000000000000000 ) ) ;
#1917=EDGE_CURVE ( 'NONE', #5125, #8805, #1025, .T. ) ;
#1931=DIRECTION ( 'NONE',  ( -0.000000000000000000, -0.000000000000000000, 1.000000000000000000 ) ) ;
#1932=LINE ( 'NONE', #6222, #12954 ) ;
#1936=VERTEX_POINT ( 'NONE', #10990 ) ;
#1942=CARTESIAN_POINT ( 'NONE',  ( 650.0000000000000000, 145.0000000000000568, -210.0000000000000000 ) ) ;
#1948=ORIENTED_EDGE ( 'NONE', *, *, #1428, .T. ) ;
#1954=EDGE_CURVE ( 'NONE', #10044, #10356, #14320, .T. ) ;
#1958=CARTESIAN_POINT ( 'NONE',  ( 629.0024986820136519, 164.6091003998119220, 210.0000119999999981 ) ) ;
#1964=ORIENTED_EDGE ( 'NONE', *, *, #8270, .T. ) ;
#1970=ORIENTED_EDGE ( 'NONE', *, *, #5113, .F. ) ;
#1971=LINE ( 'NONE', #5302, #12719 ) ;
#1975=EDGE_CURVE ( 'NONE', #1729, #6382, #7613, .T. ) ;
#1979=EDGE_CURVE ( 'NONE', #5923, #7944, #14323, .T. ) ;
#1985=CARTESIAN_POINT ( 'NONE',  ( 455.5035746174796714, 294.6698471414878782, -210.0000000000000000 ) ) ;
#1991=CARTESIAN_POINT ( 'NONE',  ( 642.5000000000001137, 160.0000000000000284, -210.0000119999999981 ) ) ;
#1993=DIRECTION ( 'NONE',  ( -0.2873478855663453846, -0.9578262852211513190, -0.000000000000000000 ) ) ;
#1994=ORIENTED_EDGE ( 'NONE', *, *, #8065, .T. ) ;
#1996=CARTESIAN_POINT ( 'NONE',  ( -10.00000000000000000, 413.4403065089105667, 190.0000000000000000 ) ) ;
#2013=ORIENTED_EDGE ( 'NONE', *, *, #3123, .F. ) ;
#2018=DIRECTION ( 'NONE',  ( -1.000000000000000000, 0.000000000000000000, 0.000000000000000000 ) ) ;
#2019=CARTESIAN_POINT ( 'NONE',  ( 650.0000000000000000, 145.0000000000000568, 210.0000000000000000 ) ) ;
#2032=CARTESIAN_POINT ( 'NONE',  ( -10.00000000000000000, 10.00000000000000178, -210.0020000000000095 ) ) ;
#2042=CARTESIAN_POINT ( 'NONE',  ( 631.2115189223973175, 153.4514063374357136, -210.0000000000000000 ) ) ;
#2047=LINE ( 'NONE', #12096, #5443 ) ;
#2056=AXIS2_PLACEMENT_3D ( 'NONE', #3071, #2993, #6470 ) ;
#2061=DIRECTION ( 'NONE',  ( 0.000000000000000000, -0.000000000000000000, -1.000000000000000000 ) ) ;
#2064=ORIENTED_EDGE ( 'NONE', *, *, #13825, .F. ) ;
#2078=AXIS2_PLACEMENT_3D ( 'NONE', #2287, #9161, #10046 ) ;
#2084=ORIENTED_EDGE ( 'NONE', *, *, #5673, .F. ) ;
#2098=ORIENTED_EDGE ( 'NONE', *, *, #2675, .T. ) ;
#2099=CIRCLE ( 'NONE', #10360, 5.249999999999976907 ) ;
#2100=DIRECTION ( 'NONE',  ( 0.000000000000000000, 1.000000000000000000, 0.000000000000000000 ) ) ;
#2103=ORIENTED_EDGE ( 'NONE', *, *, #9085, .F. ) ;
#2116=AXIS2_PLACEMENT_3D ( 'NONE', #8413, #3866, #12925 ) ;
#2117=CARTESIAN_POINT ( 'NONE',  ( 633.0482295921264040, 152.6904006748949030, -210.0000000000000000 ) ) ;
#2121=DIRECTION ( 'NONE',  ( 1.000000000000000000, 0.000000000000000000, 0.000000000000000000 ) ) ;
#2130=EDGE_CURVE ( 'NONE', #7506, #3336, #2792, .T. ) ;
#2136=EDGE_CURVE ( 'NONE', #9276, #4023, #8328, .T. ) ;
#2142=AXIS2_PLACEMENT_3D ( 'NONE', #6346, #7746, #2121 ) ;
#2157=ORIENTED_EDGE ( 'NONE', *, *, #4058, .T. ) ;
#2161=EDGE_CURVE ( 'NONE', #10356, #7765, #6200, .T. ) ;
#2167=FACE_OUTER_BOUND ( 'NONE', #3892, .T. ) ;
#2176=CARTESIAN_POINT ( 'NONE',  ( 10.00000000000000000, 0.000000000000000000, -210.0000000000000000 ) ) ;
#2177=ORIENTED_EDGE ( 'NONE', *, *, #1917, .F. ) ;
#2184=LINE ( 'NONE', #11038, #10409 ) ;
#2185=CIRCLE ( 'NONE', #2668, 2.649999999999985700 ) ;
#2197=DIRECTION ( 'NONE',  ( -1.000000000000000000, 0.000000000000000000, 0.000000000000000000 ) ) ;
#2203=LINE ( 'NONE', #6930, #324 ) ;
#2207=EDGE_CURVE ( 'NONE', #9473, #1845, #8475, .T. ) ;
#2237=CARTESIAN_POINT ( 'NONE',  ( 446.3084422793565409, 264.0194060144110608, 210.0000000000000000 ) ) ;
#2240=FACE_OUTER_BOUND ( 'NONE', #10042, .T. ) ;
#2241=ORIENTED_EDGE ( 'NONE', *, *, #8930, .T. ) ;
#2245=DIRECTION ( 'NONE',  ( -0.000000000000000000, -0.000000000000000000, 1.000000000000000000 ) ) ;
#2250=CARTESIAN_POINT ( 'NONE',  ( 139.8040310085880833, 355.9707293956415697, 190.0000000000000000 ) ) ;
#2257=EDGE_LOOP ( 'NONE', ( #9149, #722, #9505, #994 ) ) ;
#2260=DIRECTION ( 'NONE',  ( 0.000000000000000000, -1.000000000000000000, 0.000000000000000000 ) ) ;
#2264=EDGE_CURVE ( 'NONE', #14524, #1319, #13839, .T. ) ;
#2271=VERTEX_POINT ( 'NONE', #11908 ) ;
#2276=PLANE ( 'NONE',  #12484 ) ;
#2282=CARTESIAN_POINT ( 'NONE',  ( 153.1991633467111456, 386.6211705227183870, -210.0000000000000000 ) ) ;
#2284=VECTOR ( 'NONE', #2575, 1000.000000000000000 ) ;
#2287=CARTESIAN_POINT ( 'NONE',  ( 455.5035746174796714, 294.6698471414878782, 210.0000000000000000 ) ) ;
#2292=DIRECTION ( 'NONE',  ( 0.000000000000000000, 0.000000000000000000, -1.000000000000000000 ) ) ;
#2301=PLANE ( 'NONE',  #12720 ) ;
#2310=EDGE_CURVE ( 'NONE', #8377, #72, #7268, .T. ) ;
#2321=AXIS2_PLACEMENT_3D ( 'NONE', #7580, #10903, #9790 ) ;
#2337=CARTESIAN_POINT ( 'NONE',  ( 164.3243839102495656, 402.9042173714779551, -190.0000000000000000 ) ) ;
#2341=ADVANCED_FACE ( 'NONE', ( #384 ), #12881, .F. ) ;
#2344=ADVANCED_FACE ( 'NONE', ( #2845 ), #12814, .F. ) ;
#2354=CIRCLE ( 'NONE', #8012, 4.199999999999981526 ) ;
#2359=ORIENTED_EDGE ( 'NONE', *, *, #1975, .T. ) ;
#2375=CARTESIAN_POINT ( 'NONE',  ( 446.3084422793565409, 264.0194060144110608, 210.0000000000000000 ) ) ;
#2376=ORIENTED_EDGE ( 'NONE', *, *, #6692, .T. ) ;
#2378=VECTOR ( 'NONE', #9459, 1000.000000000000000 ) ;
#2382=AXIS2_PLACEMENT_3D ( 'NONE', #7418, #8300, #2627 ) ;
#2387=AXIS2_PLACEMENT_3D ( 'NONE', #4343, #8838, #3224 ) ;
#2390=CARTESIAN_POINT ( 'NONE',  ( -9.498873539028489220E-16, 10.00000000000000000, 210.0000000000000000 ) ) ;
#2395=ORIENTED_EDGE ( 'NONE', *, *, #5341, .F. ) ;
#2402=EDGE_LOOP ( 'NONE', ( #1994, #3074 ) ) ;
#2404=ADVANCED_FACE ( 'NONE', ( #5327 ), #1776, .F. ) ;
#2410=CARTESIAN_POINT ( 'NONE',  ( 590.0000000000000000, 10.00000000000005507, -210.0000000000000000 ) ) ;
#2411=FACE_OUTER_BOUND ( 'NONE', #1775, .T. ) ;
#2419=ORIENTED_EDGE ( 'NONE', *, *, #3611, .T. ) ;
#2442=DIRECTION ( 'NONE',  ( 1.000000000000000000, 0.000000000000000000, 0.000000000000000000 ) ) ;
#2444=CARTESIAN_POINT ( 'NONE',  ( 627.5000000000000000, 160.0000000000000284, 210.0000059999999849 ) ) ;
#2454=CARTESIAN_POINT ( 'NONE',  ( 133.6739427831727767, 370.3381236739588189, 190.0000000000000000 ) ) ;
#2460=ADVANCED_FACE ( 'NONE', ( #7460 ), #5181, .F. ) ;
#2471=CARTESIAN_POINT ( 'NONE',  ( 610.0000000000000000, 10.00000000000005507, -190.0000000000000000 ) ) ;
#2476=CARTESIAN_POINT ( 'NONE',  ( 440.1783540539411774, 278.3868002927282532, 210.0000000000000000 ) ) ;
#2477=DIRECTION ( 'NONE',  ( -0.000000000000000000, -0.000000000000000000, -1.000000000000000000 ) ) ;
#2478=ORIENTED_EDGE ( 'NONE', *, *, #13536, .F. ) ;
#2479=DIRECTION ( 'NONE',  ( 1.000000000000000000, 0.000000000000000000, -0.000000000000000000 ) ) ;
#2487=CARTESIAN_POINT ( 'NONE',  ( 459.7035746174796031, 294.6698471414878782, -210.0000000000000000 ) ) ;
#2503=ADVANCED_FACE ( 'NONE', ( #13010 ), #2739, .F. ) ;
#2504=CARTESIAN_POINT ( 'NONE',  ( 443.6584422793565636, 264.0194060144110608, 187.0000000000000000 ) ) ;
#2517=LINE ( 'NONE', #4898, #11078 ) ;
#2521=VECTOR ( 'NONE', #5896, 1000.000000000000000 ) ;
#2522=ORIENTED_EDGE ( 'NONE', *, *, #5409, .F. ) ;
#2525=ORIENTED_EDGE ( 'NONE', *, *, #12151, .T. ) ;
#2526=DIRECTION ( 'NONE',  ( -0.000000000000000000, -0.000000000000000000, 1.000000000000000000 ) ) ;
#2531=CARTESIAN_POINT ( 'NONE',  ( 0.000000000000000000, 0.000000000000000000, 190.0000000000000000 ) ) ;
#2538=AXIS2_PLACEMENT_3D ( 'NONE', #8528, #4920, #9567 ) ;
#2551=PLANE ( 'NONE',  #12307 ) ;
#2558=ORIENTED_EDGE ( 'NONE', *, *, #2136, .F. ) ;
#2559=CARTESIAN_POINT ( 'NONE',  ( 590.0000000000000000, 10.00000000000005507, 210.0000000000000000 ) ) ;
#2561=VECTOR ( 'NONE', #11667, 1000.000000000000000 ) ;
#2562=VECTOR ( 'NONE', #7394, 1000.000000000000227 ) ;
#2563=DIRECTION ( 'NONE',  ( -0.9578262852211515410, 0.2873478855663446074, -0.000000000000000000 ) ) ;
#2575=DIRECTION ( 'NONE',  ( 0.000000000000000000, 1.000000000000000000, 0.000000000000000000 ) ) ;
#2578=ORIENTED_EDGE ( 'NONE', *, *, #11158, .F. ) ;
#2582=VECTOR ( 'NONE', #12371, 1000.000000000000000 ) ;
#2597=CARTESIAN_POINT ( 'NONE',  ( 470.8287951810180516, 310.9528939902474463, -210.0000000000000000 ) ) ;
#2607=VECTOR ( 'NONE', #8502, 1000.000000000000114 ) ;
#2614=CARTESIAN_POINT ( 'NONE',  ( 164.3243839102495656, 402.9042173714779551, -190.0000000000000000 ) ) ;
#2616=DIRECTION ( 'NONE',  ( 0.9578262852211508749, -0.2873478855663467724, 0.000000000000000000 ) ) ;
#2627=DIRECTION ( 'NONE',  ( -1.000000000000000000, 0.000000000000000000, 0.000000000000000000 ) ) ;
#2635=VERTEX_POINT ( 'NONE', #12619 ) ;
#2647=LINE ( 'NONE', #12668, #11303 ) ;
#2658=ORIENTED_EDGE ( 'NONE', *, *, #10835, .T. ) ;
#2660=VERTEX_POINT ( 'NONE', #2725 ) ;
#2663=DIRECTION ( 'NONE',  ( 1.000000000000000000, 0.000000000000000000, 0.000000000000000000 ) ) ;
#2668=AXIS2_PLACEMENT_3D ( 'NONE', #14504, #3072, #14444 ) ;
#2675=EDGE_CURVE ( 'NONE', #1319, #9797, #3986, .T. ) ;
#2677=EDGE_LOOP ( 'NONE', ( #12262, #12023 ) ) ;
#2679=CARTESIAN_POINT ( 'NONE',  ( 144.7991633467111683, 386.6211705227183870, -210.0000000000000000 ) ) ;
#2682=DIRECTION ( 'NONE',  ( -0.000000000000000000, 0.000000000000000000, -1.000000000000000000 ) ) ;
#2709=DIRECTION ( 'NONE',  ( -0.9578262852211517631, 0.2873478855663438858, -0.000000000000000000 ) ) ;
#2723=EDGE_LOOP ( 'NONE', ( #11965, #3945, #5282, #12334 ) ) ;
#2725=CARTESIAN_POINT ( 'NONE',  ( 152.8304684875957662, 364.5911659626319761, -190.0000000000000000 ) ) ;
#2739=PLANE ( 'NONE',  #9855 ) ;
#2747=DIRECTION ( 'NONE',  ( -0.000000000000000000, -0.000000000000000000, 1.000000000000000000 ) ) ;
#2749=CARTESIAN_POINT ( 'NONE',  ( 164.3243839102495656, 402.9042173714779551, -210.0000000000000000 ) ) ;
#2756=ORIENTED_EDGE ( 'NONE', *, *, #10128, .T. ) ;
#2759=EDGE_CURVE ( 'NONE', #214, #503, #7739, .T. ) ;
#2761=FACE_BOUND ( 'NONE', #10258, .T. ) ;
#2768=CARTESIAN_POINT ( 'NONE',  ( 144.7991633467111399, 386.6211705227183870, 210.0000000000000000 ) ) ;
#2775=EDGE_CURVE ( 'NONE', #525, #739, #4281, .T. ) ;
#2792=LINE ( 'NONE', #4948, #2284 ) ;
#2801=VECTOR ( 'NONE', #5063, 1000.000000000000000 ) ;
#2824=ORIENTED_EDGE ( 'NONE', *, *, #2864, .F. ) ;
#2825=CARTESIAN_POINT ( 'NONE',  ( 10.00000000000000000, 386.5596934910894902, -210.0000000000000000 ) ) ;
#2832=DIRECTION ( 'NONE',  ( -0.000000000000000000, -0.000000000000000000, -1.000000000000000000 ) ) ;
#2839=DIRECTION ( 'NONE',  ( -0.9578262852211513190, 0.2873478855663453846, 0.000000000000000000 ) ) ;
#2845=FACE_OUTER_BOUND ( 'NONE', #13127, .T. ) ;
#2847=VERTEX_POINT ( 'NONE', #11053 ) ;
#2849=DIRECTION ( 'NONE',  ( 1.387778780781446464E-15, -2.775557561562892929E-15, 1.000000000000000000 ) ) ;
#2856=CIRCLE ( 'NONE', #13220, 5.249999999999976907 ) ;
#2858=DIRECTION ( 'NONE',  ( 0.000000000000000000, -1.000000000000000000, 0.000000000000000000 ) ) ;
#2862=AXIS2_PLACEMENT_3D ( 'NONE', #13566, #3536, #6927 ) ;
#2863=PLANE ( 'NONE',  #5628 ) ;
#2864=EDGE_CURVE ( 'NONE', #12665, #352, #3098, .T. ) ;
#2866=CIRCLE ( 'NONE', #5689, 4.199999999999981526 ) ;
#2868=ADVANCED_FACE ( 'NONE', ( #14385 ), #3390, .F. ) ;
#2882=ORIENTED_EDGE ( 'NONE', *, *, #13158, .F. ) ;
#2886=DIRECTION ( 'NONE',  ( -0.000000000000000000, -0.000000000000000000, -1.000000000000000000 ) ) ;
#2888=CARTESIAN_POINT ( 'NONE',  ( -10.00000000000000000, 0.000000000000000000, 210.0000000000000000 ) ) ;
#2898=STYLED_ITEM('',(#14653),#11938);
#2899=DIRECTION ( 'NONE',  ( -0.2873478855663454401, -0.9578262852211514300, 0.000000000000000000 ) ) ;
#2920=LINE ( 'NONE', #6235, #1198 ) ;
#2928=CARTESIAN_POINT ( 'NONE',  ( 642.3047950750125210, 161.9631091326946830, 210.0000120000000265 ) ) ;
#2938=CARTESIAN_POINT ( 'NONE',  ( 610.0000000000000000, 175.0000000000000568, 210.0000000000000000 ) ) ;
#2940=DIRECTION ( 'NONE',  ( 0.000000000000000000, -0.000000000000000000, -1.000000000000000000 ) ) ;
#2949=VERTEX_POINT ( 'NONE', #3451 ) ;
#2954=CARTESIAN_POINT ( 'NONE',  ( 642.5000000000001137, 160.0000000000000284, -210.0000059999999849 ) ) ;
#2973=CARTESIAN_POINT ( 'NONE',  ( 470.8287951810180516, 310.9528939902474463, -210.0000000000000000 ) ) ;
#2986=EDGE_CURVE ( 'NONE', #10129, #4375, #11351, .T. ) ;
#2989=VERTEX_POINT ( 'NONE', #258 ) ;
#2990=VERTEX_POINT ( 'NONE', #8159 ) ;
#2992=CARTESIAN_POINT ( 'NONE',  ( 638.7771423527817660, 166.5533979126570614, 210.0000120000000265 ) ) ;
#2993=DIRECTION ( 'NONE',  ( -0.000000000000000000, -0.000000000000000000, -1.000000000000000000 ) ) ;
#3008=CARTESIAN_POINT ( 'NONE',  ( 112.9652219749295341, 376.5507399164317803, 190.0000000000000000 ) ) ;
#3017=VERTEX_POINT ( 'NONE', #2559 ) ;
#3021=CARTESIAN_POINT ( 'NONE',  ( 139.8040310085880833, 355.9707293956415697, -190.0000000000000000 ) ) ;
#3036=LINE ( 'NONE', #3183, #1895 ) ;
#3041=ADVANCED_FACE ( 'NONE', ( #6186, #562, #5148, #3904, #8386, #4322 ), #2863, .F. ) ;
#3049=LINE ( 'NONE', #1855, #9272 ) ;
#3057=VECTOR ( 'NONE', #5520, 1000.000000000000000 ) ;
#3058=ORIENTED_EDGE ( 'NONE', *, *, #7142, .F. ) ;
#3071=CARTESIAN_POINT ( 'NONE',  ( 446.3084422793565409, 264.0194060144110608, -210.0000000000000000 ) ) ;
#3072=DIRECTION ( 'NONE',  ( 0.000000000000000000, 0.000000000000000000, 1.000000000000000000 ) ) ;
#3074=ORIENTED_EDGE ( 'NONE', *, *, #9191, .T. ) ;
#3076=ORIENTED_EDGE ( 'NONE', *, *, #5920, .F. ) ;
#3077=DIRECTION ( 'NONE',  ( -0.000000000000000000, -1.000000000000000000, -0.000000000000000000 ) ) ;
#3080=CARTESIAN_POINT ( 'NONE',  ( 10.00000000000000000, 10.00000000000000178, 190.0000000000000000 ) ) ;
#3084=ORIENTED_EDGE ( 'NONE', *, *, #281, .T. ) ;
#3085=LINE ( 'NONE', #3008, #13703 ) ;
#3090=SHAPE_REPRESENTATION_RELATIONSHIP ( 'NONE' , 'NONE' ,  #1873, #3907 ) ;
#3096=VECTOR ( 'NONE', #4846, 1000.000000000000000 ) ;
#3098=LINE ( 'NONE', #7889, #176 ) ;
#3099=CIRCLE ( 'NONE', #11341, 4.199999999999981526 ) ;
#3102=CARTESIAN_POINT ( 'NONE',  ( 642.3094156464453590, 161.9516943256562911, -210.0000000000000284 ) ) ;
#3115=DIRECTION ( 'NONE',  ( -0.000000000000000000, -0.000000000000000000, -1.000000000000000000 ) ) ;
#3123=EDGE_CURVE ( 'NONE', #10957, #2949, #11985, .T. ) ;
#3128=ORIENTED_EDGE ( 'NONE', *, *, #12605, .F. ) ;
#3135=EDGE_CURVE ( 'NONE', #11363, #14011, #11774, .T. ) ;
#3137=VERTEX_POINT ( 'NONE', #7213 ) ;
#3140=CARTESIAN_POINT ( 'NONE',  ( 164.3243839102495656, 402.9042173714779551, -210.0000000000000000 ) ) ;
#3143=DIRECTION ( 'NONE',  ( -0.000000000000000000, -0.000000000000000000, -1.000000000000000000 ) ) ;
#3148=DIRECTION ( 'NONE',  ( 0.2873478855663439413, 0.9578262852211518741, -0.000000000000000000 ) ) ;
#3152=VERTEX_POINT ( 'NONE', #3140 ) ;
#3160=LINE ( 'NONE', #9946, #8237 ) ;
#3170=VERTEX_POINT ( 'NONE', #14616 ) ;
#3171=ORIENTED_EDGE ( 'NONE', *, *, #6113, .F. ) ;
#3173=CARTESIAN_POINT ( 'NONE',  ( 628.4512226587627310, 156.2114428402112765, -209.9999999999999432 ) ) ;
#3180=DIRECTION ( 'NONE',  ( -0.000000000000000000, -0.000000000000000000, 1.000000000000000000 ) ) ;
#3183=CARTESIAN_POINT ( 'NONE',  ( 112.9652219749295341, 376.5507399164317803, -210.0000000000000000 ) ) ;
#3189=LINE ( 'NONE', #13584, #3293 ) ;
#3209=LINE ( 'NONE', #6606, #10371 ) ;
#3211=DIRECTION ( 'NONE',  ( -0.000000000000000000, -0.000000000000000000, -1.000000000000000000 ) ) ;
#3212=CARTESIAN_POINT ( 'NONE',  ( 446.3084422793565409, 264.0194060144110608, -210.0000000000000000 ) ) ;
#3224=DIRECTION ( 'NONE',  ( -1.000000000000000000, 0.000000000000000000, 0.000000000000000000 ) ) ;
#3234=CARTESIAN_POINT ( 'NONE',  ( 628.9938615732160088, 155.3996772905950081, -210.0000000000000000 ) ) ;
#3239=DIRECTION ( 'NONE',  ( -0.000000000000000000, -0.000000000000000000, -1.000000000000000000 ) ) ;
#3244=CARTESIAN_POINT ( 'NONE',  ( 650.0000000000000000, 145.0000000000000568, -190.0000000000000000 ) ) ;
#3253=DIRECTION ( 'NONE',  ( 1.000000000000000000, 9.498873539028489960E-17, 0.000000000000000000 ) ) ;
#3262=ORIENTED_EDGE ( 'NONE', *, *, #7448, .T. ) ;
#3265=CARTESIAN_POINT ( 'NONE',  ( 470.8287951810180516, 310.9528939902474463, -210.0000000000000000 ) ) ;
#3280=AXIS2_PLACEMENT_3D ( 'NONE', #12994, #2886, #7385 ) ;
#3286=ORIENTED_EDGE ( 'NONE', *, *, #5552, .F. ) ;
#3289=VERTEX_POINT ( 'NONE', #10280 ) ;
#3290=FACE_OUTER_BOUND ( 'NONE', #8079, .T. ) ;
#3293=VECTOR ( 'NONE', #7908, 1000.000000000000000 ) ;
#3302=CIRCLE ( 'NONE', #6367, 2.649999999999985700 ) ;
#3309=EDGE_LOOP ( 'NONE', ( #780, #9205, #13000, #1149 ) ) ;
#3310=EDGE_CURVE ( 'NONE', #4698, #10509, #3517, .T. ) ;
#3311=ORIENTED_EDGE ( 'NONE', *, *, #10418, .F. ) ;
#3313=DIRECTION ( 'NONE',  ( 1.000000000000000000, 9.498873539028489960E-17, 0.000000000000000000 ) ) ;
#3316=DIRECTION ( 'NONE',  ( 0.000000000000000000, 0.000000000000000000, 1.000000000000000000 ) ) ;
#3322=FACE_OUTER_BOUND ( 'NONE', #7315, .T. ) ;
#3326=VECTOR ( 'NONE', #6616, 1000.000000000000000 ) ;
#3330=ADVANCED_FACE ( 'NONE', ( #3575 ), #1638, .F. ) ;
#3331=VECTOR ( 'NONE', #14496, 1000.000000000000000 ) ;
#3333=CARTESIAN_POINT ( 'NONE',  ( 443.6584422793565636, 264.0194060144110608, 190.0000000000000000 ) ) ;
#3335=ORIENTED_EDGE ( 'NONE', *, *, #130, .F. ) ;
#3336=VERTEX_POINT ( 'NONE', #1561 ) ;
#3338=DIRECTION ( 'NONE',  ( -0.2873478855663453846, -0.9578262852211513190, 0.000000000000000000 ) ) ;
#3348=LINE ( 'NONE', #1942, #7742 ) ;
#3349=FACE_OUTER_BOUND ( 'NONE', #10900, .T. ) ;
#3352=PLANE ( 'NONE',  #12740 ) ;
#3358=PLANE ( 'NONE',  #4271 ) ;
#3367=DIRECTION ( 'NONE',  ( -0.000000000000000000, -0.000000000000000000, 1.000000000000000000 ) ) ;
#3368=VERTEX_POINT ( 'NONE', #7178 ) ;
#3369=DIRECTION ( 'NONE',  ( 0.000000000000000000, 0.000000000000000000, -1.000000000000000000 ) ) ;
#3371=ORIENTED_EDGE ( 'NONE', *, *, #3711, .F. ) ;
#3379=PLANE ( 'NONE',  #12518 ) ;
#3381=DIRECTION ( 'NONE',  ( 1.000000000000000000, 0.000000000000000000, 0.000000000000000000 ) ) ;
#3390=CYLINDRICAL_SURFACE ( 'NONE', #10804, 4.199999999999926459 ) ;
#3393=CARTESIAN_POINT ( 'NONE',  ( 627.6905843535678287, 158.0483056743123882, -210.0000000000000284 ) ) ;
#3396=EDGE_CURVE ( 'NONE', #11414, #54, #4679, .T. ) ;
#3407=EDGE_CURVE ( 'NONE', #54, #352, #11526, .T. ) ;
#3411=EDGE_CURVE ( 'NONE', #503, #214, #10350, .T. ) ;
#3417=DIRECTION ( 'NONE',  ( 1.000000000000000000, 0.000000000000000000, 0.000000000000000000 ) ) ;
#3436=ORIENTED_EDGE ( 'NONE', *, *, #5552, .T. ) ;
#3442=DIRECTION ( 'NONE',  ( 0.000000000000000000, 0.000000000000000000, -1.000000000000000000 ) ) ;
#3451=CARTESIAN_POINT ( 'NONE',  ( 443.6584422793565636, 264.0194060144110608, -210.0000000000000000 ) ) ;
#3470=ORIENTED_EDGE ( 'NONE', *, *, #3680, .T. ) ;
#3473=VECTOR ( 'NONE', #8121, 1000.000000000000000 ) ;
#3479=ADVANCED_FACE ( 'NONE', ( #13013 ), #813, .F. ) ;
#3486=EDGE_LOOP ( 'NONE', ( #4129, #8614, #10605, #6105 ) ) ;
#3487=ORIENTED_EDGE ( 'NONE', *, *, #34, .T. ) ;
#3488=CARTESIAN_POINT ( 'NONE',  ( 627.5000000000000000, 160.0000000000000284, -207.0000000000000000 ) ) ;
#3494=VECTOR ( 'NONE', #10879, 1000.000000000000000 ) ;
#3499=DIRECTION ( 'NONE',  ( -0.000000000000000000, -0.000000000000000000, -1.000000000000000000 ) ) ;
#3511=EDGE_CURVE ( 'NONE', #10831, #14275, #1932, .T. ) ;
#3513=AXIS2_PLACEMENT_3D ( 'NONE', #6996, #9074, #1477 ) ;
#3516=CARTESIAN_POINT ( 'NONE',  ( 629.7500000000000000, 160.0000000000000284, -190.0000000000000000 ) ) ;
#3517=CIRCLE ( 'NONE', #432, 4.199999999999926459 ) ;
#3520=DIRECTION ( 'NONE',  ( -0.000000000000000000, 0.000000000000000000, -1.000000000000000000 ) ) ;
#3523=DIRECTION ( 'NONE',  ( -1.000000000000000000, 0.000000000000000000, 0.000000000000000000 ) ) ;
#3535=LINE ( 'NONE', #104, #484 ) ;
#3536=DIRECTION ( 'NONE',  ( -0.9578262852211514300, 0.2873478855663454401, 0.000000000000000000 ) ) ;
#3540=CARTESIAN_POINT ( 'NONE',  ( 124.4591373975826230, 414.8637913252775888, 0.000000000000000000 ) ) ;
#3553=CARTESIAN_POINT ( 'NONE',  ( -9.498873539028489220E-16, 10.00000000000000000, 210.0000000000000000 ) ) ;
#3561=UNCERTAINTY_MEASURE_WITH_UNIT (LENGTH_MEASURE( 1.000000000000000082E-05 ), #1076, 'distance_accuracy_value', 'NONE');
#3570=ORIENTED_EDGE ( 'NONE', *, *, #12241, .F. ) ;
#3572=CARTESIAN_POINT ( 'NONE',  ( 629.0024986820135382, 155.3908996001881064, 210.0000120000000265 ) ) ;
#3575=FACE_OUTER_BOUND ( 'NONE', #12948, .T. ) ;
#3579=CYLINDRICAL_SURFACE ( 'NONE', #3803, 5.249999999999976907 ) ;
#3583=CARTESIAN_POINT ( 'NONE',  ( 0.000000000000000000, 0.000000000000000000, -210.0000000000000000 ) ) ;
#3598=CARTESIAN_POINT ( 'NONE',  ( 459.3348797583643091, 272.6398425814014104, 210.0000000000000000 ) ) ;
#3611=EDGE_CURVE ( 'NONE', #14241, #10194, #3189, .T. ) ;
#3614=ORIENTED_EDGE ( 'NONE', *, *, #7142, .T. ) ;
#3618=ORIENTED_EDGE ( 'NONE', *, *, #1979, .T. ) ;
#3621=PLANE ( 'NONE',  #10386 ) ;
#3637=EDGE_CURVE ( 'NONE', #145, #7099, #11220, .T. ) ;
#3644=CARTESIAN_POINT ( 'NONE',  ( -10.00000000000000000, 10.00000000000000178, -190.0000000000000000 ) ) ;
#3652=AXIS2_PLACEMENT_3D ( 'NONE', #4425, #6712, #8923 ) ;
#3655=CARTESIAN_POINT ( 'NONE',  ( 145.1678582058265476, 408.6511750828048548, 190.0000000000000000 ) ) ;
#3657=DIRECTION ( 'NONE',  ( 1.000000000000000000, 9.498873539028489960E-17, 0.000000000000000000 ) ) ;
#3658=DIRECTION ( 'NONE',  ( -0.000000000000000000, -0.000000000000000000, -1.000000000000000000 ) ) ;
#3659=ADVANCED_FACE ( 'NONE', ( #881 ), #8865, .F. ) ;
#3663=ORIENTED_EDGE ( 'NONE', *, *, #11458, .F. ) ;
#3670=CARTESIAN_POINT ( 'NONE',  ( 448.9584422793565750, 264.0194060144110608, 210.0000000000000000 ) ) ;
#3680=EDGE_CURVE ( 'NONE', #3017, #14524, #1181, .T. ) ;
#3686=EDGE_CURVE ( 'NONE', #13114, #8286, #4436, .T. ) ;
#3697=ORIENTED_EDGE ( 'NONE', *, *, #493, .T. ) ;
#3711=EDGE_CURVE ( 'NONE', #5965, #12303, #8116, .T. ) ;
#3713=CIRCLE ( 'NONE', #1818, 4.200000000000009059 ) ;
#3715=EDGE_LOOP ( 'NONE', ( #10104, #12863, #363, #4291 ) ) ;
#3736=PLANE ( 'NONE',  #10851 ) ;
#3761=CYLINDRICAL_SURFACE ( 'NONE', #10195, 5.249999999999976907 ) ;
#3764=B_SPLINE_CURVE_WITH_KNOTS ( 'NONE', 3,
 ( #14311, #1763, #3102, #10766, #14179, #646, #14528, #11203, #5464, #6851, #12308, #11057, #1085, #938, #5675, #9881, #1017, #13420 ),
 .UNSPECIFIED., .F., .F.,
 ( 4, 2, 2, 2, 2, 2, 2, 2, 4 ),
 ( 0.5000000000000000000, 0.5625000000000000000, 0.6250000000000000000, 0.6875000000000000000, 0.7500000000000000000, 0.8125000000000000000, 0.8750000000000000000, 0.9375000000000000000, 1.000000000000000000 ),
 .UNSPECIFIED. ) ;
#3768=DIRECTION ( 'NONE',  ( 0.000000000000000000, -1.000000000000000000, 0.000000000000000000 ) ) ;
#3778=VECTOR ( 'NONE', #2260, 1000.000000000000000 ) ;
#3780=DIRECTION ( 'NONE',  ( 0.000000000000000000, 0.000000000000000000, -1.000000000000000000 ) ) ;
#3792=EDGE_CURVE ( 'NONE', #10509, #4698, #11059, .T. ) ;
#3795=EDGE_LOOP ( 'NONE', ( #257, #14445, #417, #4368 ) ) ;
#3801=VECTOR ( 'NONE', #7457, 1000.000000000000000 ) ;
#3803=AXIS2_PLACEMENT_3D ( 'NONE', #8068, #4960, #2 ) ;
#3805=CARTESIAN_POINT ( 'NONE',  ( 650.0000000000000000, 175.0000000000000568, -190.0000000000000000 ) ) ;
#3814=PLANE ( 'NONE',  #1658 ) ;
#3818=AXIS2_PLACEMENT_3D ( 'NONE', #6831, #11625, #13775 ) ;
#3821=VECTOR ( 'NONE', #980, 1000.000000000000000 ) ;
#3831=ORIENTED_EDGE ( 'NONE', *, *, #10608, .T. ) ;
#3832=VECTOR ( 'NONE', #6698, 1000.000000000000000 ) ;
#3857=CARTESIAN_POINT ( 'NONE',  ( -10.00000000000000000, 10.00000000000000178, 190.0000000000000000 ) ) ;
#3858=VECTOR ( 'NONE', #2832, 1000.000000000000000 ) ;
#3866=DIRECTION ( 'NONE',  ( 0.000000000000000000, 0.000000000000000000, -1.000000000000000000 ) ) ;
#3871=DIRECTION ( 'NONE',  ( 1.000000000000000000, 0.000000000000000000, -0.000000000000000000 ) ) ;
#3878=LINE ( 'NONE', #300, #10656 ) ;
#3886=ORIENTED_EDGE ( 'NONE', *, *, #5739, .F. ) ;
#3892=EDGE_LOOP ( 'NONE', ( #11616, #5955, #4440, #10151, #4414, #10675, #8349, #5616, #3915, #10949, #3663, #10239, #8668, #1673, #12573, #3128 ) ) ;
#3898=ADVANCED_FACE ( 'NONE', ( #10925 ), #7447, .F. ) ;
#3903=B_SPLINE_CURVE_WITH_KNOTS ( 'NONE', 3,
 ( #4284, #13282, #3393, #3173, #3234, #7676, #2042, #2117, #4722, #5809, #11420, #1244, #9130, #10394, #11484, #1379, #103, #8028 ),
 .UNSPECIFIED., .F., .F.,
 ( 4, 2, 2, 2, 2, 2, 2, 2, 4 ),
 ( 0.000000000000000000, 0.06250000000000000000, 0.1250000000000000000, 0.1875000000000000000, 0.2500000000000000000, 0.3125000000000000000, 0.3750000000000000000, 0.4375000000000000000, 0.5000000000000000000 ),
 .UNSPECIFIED. ) ;
#3904=FACE_BOUND ( 'NONE', #7831, .T. ) ;
#3907=ADVANCED_BREP_SHAPE_REPRESENTATION ( '', ( #11938, #9440 ), #7553 ) ;
#3911=LINE ( 'NONE', #9664, #13924 ) ;
#3913=ORIENTED_EDGE ( 'NONE', *, *, #2775, .T. ) ;
#3915=ORIENTED_EDGE ( 'NONE', *, *, #3135, .F. ) ;
#3921=CARTESIAN_POINT ( 'NONE',  ( -9.498873539028489220E-16, 10.00000000000000000, 190.0000000000000000 ) ) ;
#3922=DIRECTION ( 'NONE',  ( -0.000000000000000000, -0.000000000000000000, 1.000000000000000000 ) ) ;
#3929=ORIENTED_EDGE ( 'NONE', *, *, #5456, .F. ) ;
#3938=ADVANCED_FACE ( 'NONE', ( #5099 ), #8482, .F. ) ;
#3945=ORIENTED_EDGE ( 'NONE', *, *, #9548, .F. ) ;
#3952=DIRECTION ( 'NONE',  ( 1.000000000000000000, 0.000000000000000000, 0.000000000000000000 ) ) ;
#3960=EDGE_CURVE ( 'NONE', #3137, #1936, #8915, .T. ) ;
#3964=CARTESIAN_POINT ( 'NONE',  ( 470.8287951810180516, 310.9528939902474463, -210.0000000000000000 ) ) ;
#3968=EDGE_CURVE ( 'NONE', #13396, #7052, #5879, .T. ) ;
#3972=AXIS2_PLACEMENT_3D ( 'NONE', #14193, #11819, #8350 ) ;
#3986=LINE ( 'NONE', #7228, #6326 ) ;
#3990=LINE ( 'NONE', #3857, #14392 ) ;
#4003=DIRECTION ( 'NONE',  ( -1.000000000000000000, 0.000000000000000000, 0.000000000000000000 ) ) ;
#4004=CARTESIAN_POINT ( 'NONE',  ( 440.1783540539412343, 278.3868002927283101, -210.0000000000000000 ) ) ;
#4005=EDGE_CURVE ( 'NONE', #5821, #11723, #11054, .T. ) ;
#4018=LINE ( 'NONE', #14055, #885 ) ;
#4021=ORIENTED_EDGE ( 'NONE', *, *, #4371, .F. ) ;
#4023=VERTEX_POINT ( 'NONE', #9961 ) ;
#4025=AXIS2_PLACEMENT_3D ( 'NONE', #8257, #10482, #2663 ) ;
#4026=FACE_OUTER_BOUND ( 'NONE', #9763, .T. ) ;
#4033=ADVANCED_FACE ( 'NONE', ( #1084 ), #13208, .T. ) ;
#4034=VECTOR ( 'NONE', #6135, 1000.000000000000000 ) ;
#4042=VECTOR ( 'NONE', #8819, 1000.000000000000000 ) ;
#4058=EDGE_CURVE ( 'NONE', #5634, #13901, #6641, .T. ) ;
#4082=DIRECTION ( 'NONE',  ( 0.9578262852211513190, -0.2873478855663453846, 0.000000000000000000 ) ) ;
#4089=EDGE_CURVE ( 'NONE', #10470, #5125, #3903, .T. ) ;
#4100=EDGE_CURVE ( 'NONE', #902, #3137, #261, .T. ) ;
#4104=EDGE_LOOP ( 'NONE', ( #2064, #12090, #5796, #4473 ) ) ;
#4107=ORIENTED_EDGE ( 'NONE', *, *, #9548, .T. ) ;
#4110=ORIENTED_EDGE ( 'NONE', *, *, #6080, .T. ) ;
#4111=ORIENTED_EDGE ( 'NONE', *, *, #5612, .F. ) ;
#4113=EDGE_CURVE ( 'NONE', #72, #2660, #6985, .T. ) ;
#4114=CARTESIAN_POINT ( 'NONE',  ( 627.5000000000000000, 160.9817477042468283, 210.0000120000000265 ) ) ;
#4128=LINE ( 'NONE', #850, #10201 ) ;
#4129=ORIENTED_EDGE ( 'NONE', *, *, #4466, .F. ) ;
#4135=EDGE_CURVE ( 'NONE', #6803, #12905, #2647, .T. ) ;
#4138=CARTESIAN_POINT ( 'NONE',  ( 635.0000000000000000, 160.0000000000000284, -210.0000000000000000 ) ) ;
#4153=CARTESIAN_POINT ( 'NONE',  ( 139.8040310085880833, 355.9707293956415697, 210.0000000000000000 ) ) ;
#4154=DIRECTION ( 'NONE',  ( 0.000000000000000000, 0.000000000000000000, 1.000000000000000000 ) ) ;
#4168=DIRECTION ( 'NONE',  ( -0.000000000000000000, -0.000000000000000000, 1.000000000000000000 ) ) ;
#4181=PLANE ( 'NONE',  #988 ) ;
#4182=VECTOR ( 'NONE', #8409, 1000.000000000000000 ) ;
#4195=CARTESIAN_POINT ( 'NONE',  ( 107.2182642636026202, 357.3942142120087055, -210.0000000000000000 ) ) ;
#4222=LINE ( 'NONE', #14330, #6847 ) ;
#4224=AXIS2_PLACEMENT_3D ( 'NONE', #7025, #3871, #2682 ) ;
#4226=CARTESIAN_POINT ( 'NONE',  ( 650.0000000000000000, 175.0000000000000568, 210.0000000000000000 ) ) ;
#4233=LINE ( 'NONE', #13453, #3494 ) ;
#4242=CARTESIAN_POINT ( 'NONE',  ( 470.8287951810180516, 310.9528939902474463, 210.0000000000000000 ) ) ;
#4249=FACE_BOUND ( 'NONE', #7347, .T. ) ;
#4265=CIRCLE ( 'NONE', #1437, 2.649999999999985700 ) ;
#4266=CIRCLE ( 'NONE', #9679, 4.200000000000009059 ) ;
#4267=LINE ( 'NONE', #8770, #9464 ) ;
#4271=AXIS2_PLACEMENT_3D ( 'NONE', #140, #13965, #5037 ) ;
#4273=PRESENTATION_STYLE_ASSIGNMENT (( #14522 ) ) ;
#4277=ORIENTED_EDGE ( 'NONE', *, *, #4714, .F. ) ;
#4281=LINE ( 'NONE', #13499, #9631 ) ;
#4284=CARTESIAN_POINT ( 'NONE',  ( 627.5000000000000000, 160.0000000000000284, -210.0000059999999849 ) ) ;
#4291=ORIENTED_EDGE ( 'NONE', *, *, #14225, .T. ) ;
#4292=FACE_OUTER_BOUND ( 'NONE', #1358, .T. ) ;
#4298=VECTOR ( 'NONE', #6911, 1000.000000000000000 ) ;
#4315=ORIENTED_EDGE ( 'NONE', *, *, #7922, .F. ) ;
#4319=EDGE_CURVE ( 'NONE', #7886, #13629, #9192, .T. ) ;
#4322=FACE_OUTER_BOUND ( 'NONE', #12634, .T. ) ;
#4324=EDGE_CURVE ( 'NONE', #352, #14524, #9514, .T. ) ;
#4328=DIRECTION ( 'NONE',  ( 0.000000000000000000, 0.000000000000000000, 1.000000000000000000 ) ) ;
#4334=ORIENTED_EDGE ( 'NONE', *, *, #3310, .F. ) ;
#4335=CARTESIAN_POINT ( 'NONE',  ( -10.00000000000000000, -10.00000000000000000, 210.0000000000000000 ) ) ;
#4340=APPLICATION_CONTEXT ( 'automotive_design' ) ;
#4341=CARTESIAN_POINT ( 'NONE',  ( -10.00000000000000000, 413.4403065089105667, -210.0000000000000000 ) ) ;
#4343=CARTESIAN_POINT ( 'NONE',  ( 446.3084422793565409, 264.0194060144110608, -190.0000000000000000 ) ) ;
#4347=CARTESIAN_POINT ( 'NONE',  ( 0.000000000000000000, 0.000000000000000000, 0.000000000000000000 ) ) ;
#4363=DIRECTION ( 'NONE',  ( -0.000000000000000000, -0.000000000000000000, 1.000000000000000000 ) ) ;
#4368=ORIENTED_EDGE ( 'NONE', *, *, #13041, .T. ) ;
#4370=DIRECTION ( 'NONE',  ( -0.000000000000000000, -0.000000000000000000, 1.000000000000000000 ) ) ;
#4371=EDGE_CURVE ( 'NONE', #11023, #11723, #11075, .T. ) ;
#4375=VERTEX_POINT ( 'NONE', #3080 ) ;
#4384=DIRECTION ( 'NONE',  ( -1.000000000000000000, 0.000000000000000000, 0.000000000000000000 ) ) ;
#4389=DIRECTION ( 'NONE',  ( -1.000000000000000000, -9.498873539028489960E-17, 0.000000000000000000 ) ) ;
#4393=FACE_OUTER_BOUND ( 'NONE', #12263, .T. ) ;
#4400=EDGE_LOOP ( 'NONE', ( #8592, #2525 ) ) ;
#4402=ORIENTED_EDGE ( 'NONE', *, *, #2759, .F. ) ;
#4414=ORIENTED_EDGE ( 'NONE', *, *, #7448, .F. ) ;
#4421=CARTESIAN_POINT ( 'NONE',  ( 148.9991633467111569, 386.6211705227183870, -210.0000000000000000 ) ) ;
#4425=CARTESIAN_POINT ( 'NONE',  ( 124.4591373975839304, 414.8637913252777025, 0.000000000000000000 ) ) ;
#4429=SHAPE_DEFINITION_REPRESENTATION ( #12775, #1873 ) ;
#4436=LINE ( 'NONE', #2504, #10591 ) ;
#4440=ORIENTED_EDGE ( 'NONE', *, *, #8034, .F. ) ;
#4446=EDGE_CURVE ( 'NONE', #14275, #9080, #1971, .T. ) ;
#4447=DIRECTION ( 'NONE',  ( -0.000000000000000000, -0.000000000000000000, -1.000000000000000000 ) ) ;
#4449=EDGE_LOOP ( 'NONE', ( #11541, #10923, #337, #8576 ) ) ;
#4454=DIRECTION ( 'NONE',  ( 0.000000000000000000, 0.000000000000000000, -1.000000000000000000 ) ) ;
#4457=ORIENTED_EDGE ( 'NONE', *, *, #10901, .F. ) ;
#4460=DIRECTION ( 'NONE',  ( -0.9578262852211513190, 0.2873478855663453846, 0.000000000000000000 ) ) ;
#4466=EDGE_CURVE ( 'NONE', #7506, #2990, #3160, .T. ) ;
#4468=CARTESIAN_POINT ( 'NONE',  ( 446.3084422793565409, 264.0194060144110608, -190.0000000000000000 ) ) ;
#4472=VECTOR ( 'NONE', #1458, 1000.000000000000000 ) ;
#4473=ORIENTED_EDGE ( 'NONE', *, *, #2986, .T. ) ;
#4476=VECTOR ( 'NONE', #7665, 1000.000000000000000 ) ;
#4504=LINE ( 'NONE', #1249, #7585 ) ;
#4545=PLANE ( 'NONE',  #8052 ) ;
#4562=DIRECTION ( 'NONE',  ( -1.000000000000000000, 0.000000000000000000, 0.000000000000000000 ) ) ;
#4565=CARTESIAN_POINT ( 'NONE',  ( 446.3084422793565409, 264.0194060144110608, 190.0000000000000000 ) ) ;
#4575=EDGE_CURVE ( 'NONE', #5821, #6071, #703, .T. ) ;
#4591=ORIENTED_EDGE ( 'NONE', *, *, #7, .F. ) ;
#4592=ORIENTED_EDGE ( 'NONE', *, *, #12142, .F. ) ;
#4601=ADVANCED_FACE ( 'NONE', ( #12587 ), #13773, .F. ) ;
#4619=LINE ( 'NONE', #8885, #776 ) ;
#4621=ORIENTED_EDGE ( 'NONE', *, *, #6573, .T. ) ;
#4622=DIRECTION ( 'NONE',  ( -1.000000000000000000, 0.000000000000000000, 0.000000000000000000 ) ) ;
#4627=DIRECTION ( 'NONE',  ( -0.2873478855663454401, -0.9578262852211514300, 0.000000000000000000 ) ) ;
#4633=CYLINDRICAL_SURFACE ( 'NONE', #13983, 2.649999999999985700 ) ;
#4664=ADVANCED_FACE ( 'NONE', ( #8010 ), #3736, .T. ) ;
#4668=DIRECTION ( 'NONE',  ( 1.000000000000000000, 9.498873539028489960E-17, 0.000000000000000000 ) ) ;
#4679=LINE ( 'NONE', #8067, #8460 ) ;
#4687=EDGE_LOOP ( 'NONE', ( #6124, #4771, #1948, #10936, #7758, #8433, #1308, #13323 ) ) ;
#4693=ORIENTED_EDGE ( 'NONE', *, *, #8621, .T. ) ;
#4698=VERTEX_POINT ( 'NONE', #6304 ) ;
#4701=AXIS2_PLACEMENT_3D ( 'NONE', #6932, #11577, #12455 ) ;
#4708=DIRECTION ( 'NONE',  ( 1.000000000000000000, 0.000000000000000000, 0.000000000000000000 ) ) ;
#4710=DIRECTION ( 'NONE',  ( -0.000000000000000000, -0.000000000000000000, 1.000000000000000000 ) ) ;
#4713=AXIS2_PLACEMENT_3D ( 'NONE', #5011, #11852, #1527 ) ;
#4714=EDGE_CURVE ( 'NONE', #8605, #13901, #10672, .T. ) ;
#4720=ORIENTED_EDGE ( 'NONE', *, *, #1326, .T. ) ;
#4722=CARTESIAN_POINT ( 'NONE',  ( 634.0059381729540746, 152.5000994061731490, -210.0000000000000000 ) ) ;
#4724=CARTESIAN_POINT ( 'NONE',  ( 610.0000000000000000, 10.00000000000005507, -210.0020000000000095 ) ) ;
#4728=VECTOR ( 'NONE', #2616, 1000.000000000000114 ) ;
#4739=AXIS2_PLACEMENT_3D ( 'NONE', #11947, #2899, #4082 ) ;
#4763=CARTESIAN_POINT ( 'NONE',  ( 642.5000000000002274, 159.0182522957532569, 210.0000120000000265 ) ) ;
#4770=VECTOR ( 'NONE', #7424, 1000.000000000000000 ) ;
#4771=ORIENTED_EDGE ( 'NONE', *, *, #8135, .F. ) ;
#4776=EDGE_CURVE ( 'NONE', #2271, #7181, #10513, .T. ) ;
#4788=DIRECTION ( 'NONE',  ( -0.000000000000000000, -0.000000000000000000, -1.000000000000000000 ) ) ;
#4789=CARTESIAN_POINT ( 'NONE',  ( 10.00000000000000000, 0.000000000000000000, 190.0000000000000000 ) ) ;
#4806=ADVANCED_FACE ( 'NONE', ( #12879, #2761 ), #6237, .T. ) ;
#4807=CARTESIAN_POINT ( 'NONE',  ( 112.9652219749295341, 376.5507399164317803, -210.0000000000000000 ) ) ;
#4809=CARTESIAN_POINT ( 'NONE',  ( 107.2182642636026202, 357.3942142120087055, -190.0000000000000000 ) ) ;
#4810=EDGE_LOOP ( 'NONE', ( #13970, #11199 ) ) ;
#4816=ORIENTED_EDGE ( 'NONE', *, *, #12241, .T. ) ;
#4829=CARTESIAN_POINT ( 'NONE',  ( 628.4466020873429670, 156.2228576472182056, 210.0000119999999981 ) ) ;
#4834=ORIENTED_EDGE ( 'NONE', *, *, #4089, .F. ) ;
#4838=LINE ( 'NONE', #536, #2801 ) ;
#4841=AXIS2_PLACEMENT_3D ( 'NONE', #6431, #10771, #13213 ) ;
#4844=ORIENTED_EDGE ( 'NONE', *, *, #3123, .T. ) ;
#4846=DIRECTION ( 'NONE',  ( -0.000000000000000000, -0.000000000000000000, 1.000000000000000000 ) ) ;
#4861=VERTEX_POINT ( 'NONE', #5558 ) ;
#4866=ADVANCED_FACE ( 'NONE', ( #11173 ), #5284, .F. ) ;
#4876=PLANE ( 'NONE',  #4701 ) ;
#4894=AXIS2_PLACEMENT_3D ( 'NONE', #5134, #14135, #3952 ) ;
#4897=CARTESIAN_POINT ( 'NONE',  ( 639.6091003998118367, 154.0024986820136235, 210.0000119999999981 ) ) ;
#4898=CARTESIAN_POINT ( 'NONE',  ( 650.0000000000000000, 175.0000000000000568, -190.0000000000000000 ) ) ;
#4899=DIRECTION ( 'NONE',  ( -1.000000000000000000, 0.000000000000000000, 0.000000000000000000 ) ) ;
#4903=LINE ( 'NONE', #3805, #12093 ) ;
#4905=EDGE_CURVE ( 'NONE', #9542, #11993, #14351, .T. ) ;
#4914=ORIENTED_EDGE ( 'NONE', *, *, #14113, .T. ) ;
#4920=DIRECTION ( 'NONE',  ( 0.000000000000000000, 0.000000000000000000, 1.000000000000000000 ) ) ;
#4927=CARTESIAN_POINT ( 'NONE',  ( 650.0000000000000000, 145.0000000000000568, 190.0000000000000000 ) ) ;
#4928=DIRECTION ( 'NONE',  ( 0.9578262852211513190, -0.2873478855663453846, 0.000000000000000000 ) ) ;
#4929=EDGE_LOOP ( 'NONE', ( #343, #9489, #650, #5904 ) ) ;
#4948=CARTESIAN_POINT ( 'NONE',  ( 610.0000000000000000, 0.000000000000000000, -210.0000000000000000 ) ) ;
#4949=ORIENTED_EDGE ( 'NONE', *, *, #13390, .T. ) ;
#4950=EDGE_CURVE ( 'NONE', #14014, #10129, #9926, .T. ) ;
#4960=DIRECTION ( 'NONE',  ( -0.000000000000000000, -0.000000000000000000, 1.000000000000000000 ) ) ;
#4963=DIRECTION ( 'NONE',  ( 1.000000000000000000, 9.498873539028489960E-17, 0.000000000000000000 ) ) ;
#4971=DIRECTION ( 'NONE',  ( 0.000000000000000000, -1.000000000000000000, 0.000000000000000000 ) ) ;
#4985=LINE ( 'NONE', #3655, #12979 ) ;
#4998=ADVANCED_FACE ( 'NONE', ( #10281, #9457 ), #3358, .F. ) ;
#5000=VECTOR ( 'NONE', #11782, 1000.000000000000114 ) ;
#5003=CARTESIAN_POINT ( 'NONE',  ( 142.4540310085880606, 355.9707293956415697, 210.0000000000000000 ) ) ;
#5005=ORIENTED_EDGE ( 'NONE', *, *, #11131, .F. ) ;
#5010=EDGE_LOOP ( 'NONE', ( #1398, #3487, #13533, #12472 ) ) ;
#5011=CARTESIAN_POINT ( 'NONE',  ( 0.000000000000000000, 0.000000000000000000, 190.0000000000000000 ) ) ;
#5012=DIRECTION ( 'NONE',  ( -0.9578262852211514300, 0.2873478855663454401, 0.000000000000000000 ) ) ;
#5017=ADVANCED_FACE ( 'NONE', ( #10135 ), #3579, .F. ) ;
#5020=CARTESIAN_POINT ( 'NONE',  ( 590.0000000000000000, 0.000000000000000000, -210.0000000000000000 ) ) ;
#5037=DIRECTION ( 'NONE',  ( -1.000000000000000000, -9.498873539028489960E-17, 0.000000000000000000 ) ) ;
#5048=FACE_OUTER_BOUND ( 'NONE', #3309, .T. ) ;
#5049=ORIENTED_EDGE ( 'NONE', *, *, #11337, .T. ) ;
#5050=ORIENTED_EDGE ( 'NONE', *, *, #12056, .F. ) ;
#5054=FACE_OUTER_BOUND ( 'NONE', #6181, .T. ) ;
#5063=DIRECTION ( 'NONE',  ( -0.000000000000000000, -0.000000000000000000, -1.000000000000000000 ) ) ;
#5066=ORIENTED_EDGE ( 'NONE', *, *, #4446, .F. ) ;
#5088=LINE ( 'NONE', #9363, #7840 ) ;
#5090=CARTESIAN_POINT ( 'NONE',  ( 139.8040310085880833, 355.9707293956415697, -210.0000000000000000 ) ) ;
#5099=FACE_OUTER_BOUND ( 'NONE', #7075, .T. ) ;
#5106=CARTESIAN_POINT ( 'NONE',  ( 145.1678582058265476, 408.6511750828048548, 190.0000000000000000 ) ) ;
#5108=DIRECTION ( 'NONE',  ( 0.9578262852211513190, -0.2873478855663453846, 0.000000000000000000 ) ) ;
#5110=EDGE_LOOP ( 'NONE', ( #2177, #4834, #6422, #13887 ) ) ;
#5113=EDGE_CURVE ( 'NONE', #10210, #8605, #1832, .T. ) ;
#5116=ORIENTED_EDGE ( 'NONE', *, *, #13902, .F. ) ;
#5125=VERTEX_POINT ( 'NONE', #2954 ) ;
#5131=VECTOR ( 'NONE', #6123, 1000.000000000000000 ) ;
#5134=CARTESIAN_POINT ( 'NONE',  ( 635.0000000000000000, 160.0000000000000284, 207.0000000000000000 ) ) ;
#5139=CARTESIAN_POINT ( 'NONE',  ( 636.9631091326946262, 167.3047950750124642, 210.0000119999999981 ) ) ;
#5145=FACE_BOUND ( 'NONE', #2677, .T. ) ;
#5148=FACE_BOUND ( 'NONE', #153, .T. ) ;
#5155=ADVANCED_FACE ( 'NONE', ( #11802 ), #8402, .F. ) ;
#5160=EDGE_CURVE ( 'NONE', #1836, #12898, #2856, .T. ) ;
#5163=ORIENTED_EDGE ( 'NONE', *, *, #6726, .T. ) ;
#5170=EDGE_CURVE ( 'NONE', #5125, #10470, #3764, .T. ) ;
#5172=AXIS2_PLACEMENT_3D ( 'NONE', #7890, #7820, #7741 ) ;
#5173=AXIS2_PLACEMENT_3D ( 'NONE', #3964, #5012, #11429 ) ;
#5181=CYLINDRICAL_SURFACE ( 'NONE', #3972, 5.249999999999976907 ) ;
#5194=VECTOR ( 'NONE', #1054, 1000.000000000000000 ) ;
#5204=DIRECTION ( 'NONE',  ( 1.000000000000000000, 0.000000000000000000, 0.000000000000000000 ) ) ;
#5211=EDGE_CURVE ( 'NONE', #3152, #13868, #5592, .T. ) ;
#5212=VERTEX_POINT ( 'NONE', #11355 ) ;
#5214=ORIENTED_EDGE ( 'NONE', *, *, #12240, .T. ) ;
#5218=CIRCLE ( 'NONE', #235, 4.199999999999981526 ) ;
#5223=ORIENTED_EDGE ( 'NONE', *, *, #13922, .F. ) ;
#5227=LINE ( 'NONE', #6403, #11056 ) ;
#5233=VECTOR ( 'NONE', #2839, 1000.000000000000114 ) ;
#5242=FILL_AREA_STYLE ('',( #7594 ) ) ;
#5243=CIRCLE ( 'NONE', #9238, 4.199999999999926459 ) ;
#5245=DIRECTION ( 'NONE',  ( -0.9578262852211513190, 0.2873478855663453846, 0.000000000000000000 ) ) ;
#5261=LINE ( 'NONE', #13291, #3801 ) ;
#5263=ORIENTED_EDGE ( 'NONE', *, *, #5170, .T. ) ;
#5268=AXIS2_PLACEMENT_3D ( 'NONE', #3212, #11913, #1804 ) ;
#5269=CYLINDRICAL_SURFACE ( 'NONE', #11060, 2.649999999999985700 ) ;
#5270=ORIENTED_EDGE ( 'NONE', *, *, #8099, .T. ) ;
#5272=CARTESIAN_POINT ( 'NONE',  ( 610.0000000000000000, 175.0000000000000568, 210.0000000000000000 ) ) ;
#5282=ORIENTED_EDGE ( 'NONE', *, *, #6189, .F. ) ;
#5284=CYLINDRICAL_SURFACE ( 'NONE', #12257, 2.649999999999985700 ) ;
#5285=EDGE_LOOP ( 'NONE', ( #7926, #8457, #7602, #5724 ) ) ;
#5298=CARTESIAN_POINT ( 'NONE',  ( 590.0000000000000000, 0.000000000000000000, 210.0000000000000000 ) ) ;
#5302=CARTESIAN_POINT ( 'NONE',  ( 590.0000000000000000, 0.000000000000000000, -190.0000000000000000 ) ) ;
#5311=ORIENTED_EDGE ( 'NONE', *, *, #5160, .T. ) ;
#5312=EDGE_LOOP ( 'NONE', ( #10941, #7976, #10232, #3470 ) ) ;
#5317=EDGE_CURVE ( 'NONE', #8139, #3170, #11331, .T. ) ;
#5323=CARTESIAN_POINT ( 'NONE',  ( 610.0000000000000000, -9.999999999999941380, 210.0000000000000000 ) ) ;
#5326=ORIENTED_EDGE ( 'NONE', *, *, #14113, .F. ) ;
#5327=FACE_OUTER_BOUND ( 'NONE', #12769, .T. ) ;
#5332=ORIENTED_EDGE ( 'NONE', *, *, #12142, .T. ) ;
#5341=EDGE_CURVE ( 'NONE', #14108, #793, #3535, .T. ) ;
#5343=ORIENTED_EDGE ( 'NONE', *, *, #13902, .T. ) ;
#5350=ORIENTED_EDGE ( 'NONE', *, *, #10901, .T. ) ;
#5359=DIRECTION ( 'NONE',  ( -0.9578262852211514300, 0.2873478855663454401, 0.000000000000000000 ) ) ;
#5367=CARTESIAN_POINT ( 'NONE',  ( 650.0000000000000000, 175.0000000000000568, 210.0000000000000000 ) ) ;
#5368=VECTOR ( 'NONE', #10515, 1000.000000000000114 ) ;
#5369=VECTOR ( 'NONE', #12961, 1000.000000000000000 ) ;
#5371=( NAMED_UNIT ( * ) PLANE_ANGLE_UNIT ( ) SI_UNIT ( $, .RADIAN. ) );
#5375=ORIENTED_EDGE ( 'NONE', *, *, #10608, .F. ) ;
#5378=CARTESIAN_POINT ( 'NONE',  ( -10.00000000000000000, 0.000000000000000000, -210.0000000000000000 ) ) ;
#5387=ADVANCED_FACE ( 'NONE', ( #10313 ), #11637, .F. ) ;
#5409=EDGE_CURVE ( 'NONE', #2660, #13868, #5885, .T. ) ;
#5410=DIRECTION ( 'NONE',  ( -0.000000000000000000, -0.000000000000000000, -1.000000000000000000 ) ) ;
#5418=ORIENTED_EDGE ( 'NONE', *, *, #10633, .T. ) ;
#5429=FACE_BOUND ( 'NONE', #7934, .T. ) ;
#5434=AXIS2_PLACEMENT_3D ( 'NONE', #13521, #9151, #2442 ) ;
#5436=AXIS2_PLACEMENT_3D ( 'NONE', #2176, #10149, #236 ) ;
#5443=VECTOR ( 'NONE', #6497, 1000.000000000000000 ) ;
#5445=DIRECTION ( 'NONE',  ( -1.000000000000000000, 0.000000000000000000, 0.000000000000000000 ) ) ;
#5449=AXIS2_PLACEMENT_3D ( 'NONE', #4724, #10529, #9215 ) ;
#5456=EDGE_CURVE ( 'NONE', #10831, #10448, #8685, .T. ) ;
#5464=CARTESIAN_POINT ( 'NONE',  ( 635.9940618270015875, 167.4999005938269079, -210.0000000000000000 ) ) ;
#5465=AXIS2_PLACEMENT_3D ( 'NONE', #7927, #11319, #12416 ) ;
#5483=ORIENTED_EDGE ( 'NONE', *, *, #3310, .T. ) ;
#5488=DIRECTION ( 'NONE',  ( -1.000000000000000000, 0.000000000000000000, 0.000000000000000000 ) ) ;
#5498=EDGE_CURVE ( 'NONE', #5961, #14241, #10830, .T. ) ;
#5505=CARTESIAN_POINT ( 'NONE',  ( 629.7500000000000000, 160.0000000000000284, -210.0000000000000000 ) ) ;
#5506=CARTESIAN_POINT ( 'NONE',  ( 124.4591373975826514, 414.8637913252776457, 0.000000000000000000 ) ) ;
#5507=DIRECTION ( 'NONE',  ( 0.000000000000000000, -0.000000000000000000, 1.000000000000000000 ) ) ;
#5517=CARTESIAN_POINT ( 'NONE',  ( 635.0000000000000000, 160.0000000000000284, -210.0000119999999981 ) ) ;
#5518=VERTEX_POINT ( 'NONE', #9581 ) ;
#5520=DIRECTION ( 'NONE',  ( -1.000000000000000000, -0.000000000000000000, -0.000000000000000000 ) ) ;
#5539=VERTEX_POINT ( 'NONE', #1750 ) ;
#5540=ORIENTED_EDGE ( 'NONE', *, *, #9620, .F. ) ;
#5542=DIRECTION ( 'NONE',  ( -0.9578262852211514300, 0.2873478855663454401, 0.000000000000000000 ) ) ;
#5551=VECTOR ( 'NONE', #1407, 1000.000000000000000 ) ;
#5552=EDGE_CURVE ( 'NONE', #1836, #5769, #7502, .T. ) ;
#5554=VERTEX_POINT ( 'NONE', #10910 ) ;
#5558=CARTESIAN_POINT ( 'NONE',  ( 152.8304684875957662, 364.5911659626319761, 210.0000000000000000 ) ) ;
#5561=ORIENTED_EDGE ( 'NONE', *, *, #8621, .F. ) ;
#5569=EDGE_CURVE ( 'NONE', #8728, #11174, #2866, .T. ) ;
#5570=CARTESIAN_POINT ( 'NONE',  ( 164.3243839102495656, 402.9042173714779551, 190.0000000000000000 ) ) ;
#5572=ORIENTED_EDGE ( 'NONE', *, *, #4113, .F. ) ;
#5574=ADVANCED_FACE ( 'NONE', ( #11122 ), #1003, .F. ) ;
#5575=ORIENTED_EDGE ( 'NONE', *, *, #1146, .T. ) ;
#5584=ORIENTED_EDGE ( 'NONE', *, *, #3407, .F. ) ;
#5587=EDGE_LOOP ( 'NONE', ( #8626, #7292 ) ) ;
#5589=ORIENTED_EDGE ( 'NONE', *, *, #8262, .T. ) ;
#5591=CARTESIAN_POINT ( 'NONE',  ( 107.2182642636026202, 357.3942142120087055, -210.0000000000000000 ) ) ;
#5592=LINE ( 'NONE', #41, #7566 ) ;
#5596=CARTESIAN_POINT ( 'NONE',  ( 590.0000000000000000, 212.5596934910894333, -210.0000000000000000 ) ) ;
#5612=EDGE_CURVE ( 'NONE', #6145, #13614, #6755, .T. ) ;
#5613=CARTESIAN_POINT ( 'NONE',  ( 10.00000000000000000, 10.00000000000000178, -210.0000000000000000 ) ) ;
#5616=ORIENTED_EDGE ( 'NONE', *, *, #13041, .F. ) ;
#5628=AXIS2_PLACEMENT_3D ( 'NONE', #7280, #11635, #11856 ) ;
#5633=ORIENTED_EDGE ( 'NONE', *, *, #3511, .F. ) ;
#5634=VERTEX_POINT ( 'NONE', #4341 ) ;
#5636=CARTESIAN_POINT ( 'NONE',  ( 144.7991633467111683, 386.6211705227183870, 210.0000000000000000 ) ) ;
#5637=VECTOR ( 'NONE', #4370, 1000.000000000000000 ) ;
#5639=CARTESIAN_POINT ( 'NONE',  ( 451.6722694765949768, 316.6998517015743460, -190.0000000000000000 ) ) ;
#5653=AXIS2_PLACEMENT_3D ( 'NONE', #5090, #8169, #11642 ) ;
#5654=CARTESIAN_POINT ( 'NONE',  ( 470.8287951810180516, 310.9528939902474463, 210.0000000000000000 ) ) ;
#5655=EDGE_CURVE ( 'NONE', #8377, #1538, #4267, .T. ) ;
#5659=LINE ( 'NONE', #1073, #7526 ) ;
#5669=CIRCLE ( 'NONE', #13927, 5.249999999999976907 ) ;
#5673=EDGE_CURVE ( 'NONE', #6493, #739, #2184, .T. ) ;
#5675=CARTESIAN_POINT ( 'NONE',  ( 628.4515058436089703, 163.7887212390026832, -210.0000000000000284 ) ) ;
#5676=ADVANCED_FACE ( 'NONE', ( #13485 ), #3379, .F. ) ;
#5677=PLANE ( 'NONE',  #2862 ) ;
#5686=DIRECTION ( 'NONE',  ( -0.2873478855663453846, -0.9578262852211513190, -0.000000000000000000 ) ) ;
#5689=AXIS2_PLACEMENT_3D ( 'NONE', #21, #10078, #4562 ) ;
#5691=ORIENTED_EDGE ( 'NONE', *, *, #10068, .F. ) ;
#5695=DIRECTION ( 'NONE',  ( -0.000000000000000000, -0.000000000000000000, -1.000000000000000000 ) ) ;
#5696=CIRCLE ( 'NONE', #2387, 2.649999999999985700 ) ;
#5699=DIRECTION ( 'NONE',  ( 0.000000000000000000, 1.000000000000000000, 0.000000000000000000 ) ) ;
#5704=LINE ( 'NONE', #3265, #14386 ) ;
#5707=DIRECTION ( 'NONE',  ( -1.000000000000000000, 0.000000000000000000, 0.000000000000000000 ) ) ;
#5718=DIRECTION ( 'NONE',  ( -0.000000000000000000, -0.000000000000000000, -1.000000000000000000 ) ) ;
#5721=VERTEX_POINT ( 'NONE', #5654 ) ;
#5724=ORIENTED_EDGE ( 'NONE', *, *, #918, .T. ) ;
#5729=DIRECTION ( 'NONE',  ( -0.000000000000000000, -0.000000000000000000, 1.000000000000000000 ) ) ;
#5730=ORIENTED_EDGE ( 'NONE', *, *, #14063, .T. ) ;
#5739=EDGE_CURVE ( 'NONE', #7944, #5923, #3099, .T. ) ;
#5745=EDGE_CURVE ( 'NONE', #14275, #1794, #313, .T. ) ;
#5751=CARTESIAN_POINT ( 'NONE',  ( 642.5000000000001137, 160.0000000000000284, 207.0000000000000000 ) ) ;
#5752=ORIENTED_EDGE ( 'NONE', *, *, #34, .F. ) ;
#5769=VERTEX_POINT ( 'NONE', #3516 ) ;
#5773=ORIENTED_EDGE ( 'NONE', *, *, #4319, .T. ) ;
#5774=ORIENTED_EDGE ( 'NONE', *, *, #322, .F. ) ;
#5775=CARTESIAN_POINT ( 'NONE',  ( 627.5000000000000000, 159.0182522957532285, 210.0000119999999981 ) ) ;
#5793=ADVANCED_FACE ( 'NONE', ( #12431 ), #1297, .F. ) ;
#5796=ORIENTED_EDGE ( 'NONE', *, *, #4950, .T. ) ;
#5797=DIRECTION ( 'NONE',  ( 1.000000000000000000, 0.000000000000000000, -0.000000000000000000 ) ) ;
#5803=PLANE ( 'NONE',  #8714 ) ;
#5809=CARTESIAN_POINT ( 'NONE',  ( 635.9940618270459254, 152.4999005938267658, -210.0000000000000000 ) ) ;
#5821=VERTEX_POINT ( 'NONE', #13620 ) ;
#5824=EDGE_CURVE ( 'NONE', #6382, #14559, #11336, .T. ) ;
#5832=ORIENTED_EDGE ( 'NONE', *, *, #1335, .T. ) ;
#5837=DIRECTION ( 'NONE',  ( -0.2873478855663453846, -0.9578262852211513190, -0.000000000000000000 ) ) ;
#5842=CARTESIAN_POINT ( 'NONE',  ( 144.7991633467111683, 386.6211705227183870, 190.0000000000000000 ) ) ;
#5846=AXIS2_PLACEMENT_3D ( 'NONE', #12044, #5488, #6374 ) ;
#5852=LINE ( 'NONE', #5939, #11264 ) ;
#5853=FACE_OUTER_BOUND ( 'NONE', #11638, .T. ) ;
#5864=VECTOR ( 'NONE', #5245, 1000.000000000000114 ) ;
#5870=ORIENTED_EDGE ( 'NONE', *, *, #10207, .T. ) ;
#5872=DIRECTION ( 'NONE',  ( 0.9578262852211514300, -0.2873478855663454401, 2.126801590887410810E-15 ) ) ;
#5874=( NAMED_UNIT ( * ) PLANE_ANGLE_UNIT ( ) SI_UNIT ( $, .RADIAN. ) );
#5879=CIRCLE ( 'NONE', #5172, 2.649999999999985700 ) ;
#5885=LINE ( 'NONE', #10395, #1444 ) ;
#5886=ORIENTED_EDGE ( 'NONE', *, *, #2310, .F. ) ;
#5889=VECTOR ( 'NONE', #2849, 1000.000000000000000 ) ;
#5891=DIRECTION ( 'NONE',  ( 0.2873478855663439413, 0.9578262852211518741, 0.000000000000000000 ) ) ;
#5894=ORIENTED_EDGE ( 'NONE', *, *, #5824, .T. ) ;
#5895=FACE_OUTER_BOUND ( 'NONE', #517, .T. ) ;
#5896=DIRECTION ( 'NONE',  ( -0.000000000000000000, -0.000000000000000000, -1.000000000000000000 ) ) ;
#5904=ORIENTED_EDGE ( 'NONE', *, *, #1954, .T. ) ;
#5909=AXIS2_PLACEMENT_3D ( 'NONE', #13743, #11441, #8053 ) ;
#5915=ORIENTED_EDGE ( 'NONE', *, *, #13577, .F. ) ;
#5920=EDGE_CURVE ( 'NONE', #3289, #14092, #6174, .T. ) ;
#5923=VERTEX_POINT ( 'NONE', #473 ) ;
#5928=EDGE_CURVE ( 'NONE', #793, #5539, #11239, .T. ) ;
#5939=CARTESIAN_POINT ( 'NONE',  ( 142.4540310085880606, 355.9707293956415697, -210.0000000000000000 ) ) ;
#5940=DIRECTION ( 'NONE',  ( -0.9578262852211513190, 0.2873478855663453846, 0.000000000000000000 ) ) ;
#5955=ORIENTED_EDGE ( 'NONE', *, *, #4058, .F. ) ;
#5959=LINE ( 'NONE', #2019, #529 ) ;
#5961=VERTEX_POINT ( 'NONE', #8439 ) ;
#5965=VERTEX_POINT ( 'NONE', #5003 ) ;
#5973=CARTESIAN_POINT ( 'NONE',  ( 650.0000000000000000, 145.0000000000000568, -210.0000000000000000 ) ) ;
#5984=EDGE_CURVE ( 'NONE', #12898, #1836, #10779, .T. ) ;
#5988=LINE ( 'NONE', #11659, #4182 ) ;
#5992=VECTOR ( 'NONE', #6196, 1000.000000000000000 ) ;
#5995=CARTESIAN_POINT ( 'NONE',  ( 627.5000000000000000, 160.0000000000000284, 210.0000059999999849 ) ) ;
#6026=ORIENTED_EDGE ( 'NONE', *, *, #4324, .T. ) ;
#6032=LINE ( 'NONE', #10532, #5000 ) ;
#6046=CARTESIAN_POINT ( 'NONE',  ( 455.5035746174796714, 294.6698471414878782, -190.0000000000000000 ) ) ;
#6050=CARTESIAN_POINT ( 'NONE',  ( 610.0000000000000000, 227.4403065089105951, 210.0000000000000000 ) ) ;
#6068=CARTESIAN_POINT ( 'NONE',  ( 139.8040310085880833, 355.9707293956415697, -210.0000000000000000 ) ) ;
#6071=VERTEX_POINT ( 'NONE', #5842 ) ;
#6073=EDGE_CURVE ( 'NONE', #10509, #10228, #13819, .T. ) ;
#6074=CARTESIAN_POINT ( 'NONE',  ( 590.0000000000000000, -9.999999999999941380, -190.0000000000000000 ) ) ;
#6080=EDGE_CURVE ( 'NONE', #10070, #14108, #13963, .T. ) ;
#6085=CARTESIAN_POINT ( 'NONE',  ( 133.6739427831727198, 370.3381236739588758, -210.0000000000000000 ) ) ;
#6091=DIRECTION ( 'NONE',  ( 0.2873478855663453846, 0.9578262852211513190, 0.000000000000000000 ) ) ;
#6093=CARTESIAN_POINT ( 'NONE',  ( 455.5035746174796714, 294.6698471414878782, 190.0000000000000000 ) ) ;
#6105=ORIENTED_EDGE ( 'NONE', *, *, #6303, .F. ) ;
#6113=EDGE_CURVE ( 'NONE', #8728, #5554, #11665, .T. ) ;
#6123=DIRECTION ( 'NONE',  ( -1.387778780781446464E-15, 2.775557561562892929E-15, 1.000000000000000000 ) ) ;
#6124=ORIENTED_EDGE ( 'NONE', *, *, #6692, .F. ) ;
#6135=DIRECTION ( 'NONE',  ( 0.000000000000000000, 1.000000000000000000, 0.000000000000000000 ) ) ;
#6145=VERTEX_POINT ( 'NONE', #10164 ) ;
#6165=CARTESIAN_POINT ( 'NONE',  ( 590.0000000000000000, 0.000000000000000000, -210.0000000000000000 ) ) ;
#6168=LINE ( 'NONE', #9411, #5233 ) ;
#6172=CIRCLE ( 'NONE', #11818, 7.500000000000062172 ) ;
#6174=LINE ( 'NONE', #7345, #6290 ) ;
#6176=EDGE_LOOP ( 'NONE', ( #14198, #10079, #13766, #9817 ) ) ;
#6177=PLANE ( 'NONE',  #10417 ) ;
#6181=EDGE_LOOP ( 'NONE', ( #13951, #4402, #6584, #13996 ) ) ;
#6186=FACE_BOUND ( 'NONE', #1229, .T. ) ;
#6189=EDGE_CURVE ( 'NONE', #197, #14559, #12592, .T. ) ;
#6190=DIRECTION ( 'NONE',  ( -0.000000000000000000, -0.000000000000000000, 1.000000000000000000 ) ) ;
#6196=DIRECTION ( 'NONE',  ( -1.387778780781446464E-15, 2.775557561562892929E-15, 1.000000000000000000 ) ) ;
#6200=LINE ( 'NONE', #7074, #2521 ) ;
#6206=DIRECTION ( 'NONE',  ( 0.9578262852211513190, -0.2873478855663453846, 0.000000000000000000 ) ) ;
#6213=CARTESIAN_POINT ( 'NONE',  ( -10.00000000000000000, 10.00000000000000178, 190.0000000000000000 ) ) ;
#6222=CARTESIAN_POINT ( 'NONE',  ( 590.0000000000000000, 10.00000000000005507, -210.0000000000000000 ) ) ;
#6224=ORIENTED_EDGE ( 'NONE', *, *, #5673, .T. ) ;
#6227=CARTESIAN_POINT ( 'NONE',  ( 164.3243839102495656, 402.9042173714779551, 210.0000000000000000 ) ) ;
#6230=CARTESIAN_POINT ( 'NONE',  ( 443.6584422793565636, 264.0194060144110608, -210.0000000000000000 ) ) ;
#6235=CARTESIAN_POINT ( 'NONE',  ( 451.6722694765949768, 316.6998517015743460, 190.0000000000000000 ) ) ;
#6236=EDGE_CURVE ( 'NONE', #145, #10831, #9202, .T. ) ;
#6237=PLANE ( 'NONE',  #6617 ) ;
#6242=DIRECTION ( 'NONE',  ( -0.000000000000000000, -0.000000000000000000, 1.000000000000000000 ) ) ;
#6243=CARTESIAN_POINT ( 'NONE',  ( 642.5000000000001137, 160.0000000000000284, 210.0000059999999849 ) ) ;
#6276=PLANE ( 'NONE',  #4739 ) ;
#6280=DIRECTION ( 'NONE',  ( 0.000000000000000000, 0.000000000000000000, 1.000000000000000000 ) ) ;
#6290=VECTOR ( 'NONE', #685, 1000.000000000000000 ) ;
#6293=FACE_OUTER_BOUND ( 'NONE', #7581, .T. ) ;
#6301=EDGE_CURVE ( 'NONE', #11494, #5554, #3713, .T. ) ;
#6303=EDGE_CURVE ( 'NONE', #2990, #12479, #12885, .T. ) ;
#6304=CARTESIAN_POINT ( 'NONE',  ( 459.7035746174795463, 294.6698471414878782, -190.0000000000000000 ) ) ;
#6307=CARTESIAN_POINT ( 'NONE',  ( 590.0000000000000000, 0.000000000000000000, 190.0000000000000000 ) ) ;
#6313=CARTESIAN_POINT ( 'NONE',  ( 641.5533979126568056, 163.7771423527817944, 210.0000119999999981 ) ) ;
#6326=VECTOR ( 'NONE', #9747, 1000.000000000000114 ) ;
#6327=VECTOR ( 'NONE', #5837, 1000.000000000000114 ) ;
#6338=VECTOR ( 'NONE', #2709, 1000.000000000000227 ) ;
#6340=VERTEX_POINT ( 'NONE', #4927 ) ;
#6346=CARTESIAN_POINT ( 'NONE',  ( 139.8040310085880833, 355.9707293956415697, 210.0000000000000000 ) ) ;
#6356=CARTESIAN_POINT ( 'NONE',  ( 451.3035746174797396, 294.6698471414878782, 190.0000000000000000 ) ) ;
#6358=VERTEX_POINT ( 'NONE', #3670 ) ;
#6360=DIRECTION ( 'NONE',  ( 1.000000000000000000, 0.000000000000000000, 0.000000000000000000 ) ) ;
#6361=AXIS2_PLACEMENT_3D ( 'NONE', #11999, #2245, #7725 ) ;
#6367=AXIS2_PLACEMENT_3D ( 'NONE', #4468, #3369, #4622 ) ;
#6371=ORIENTED_EDGE ( 'NONE', *, *, #9772, .T. ) ;
#6374=DIRECTION ( 'NONE',  ( 0.000000000000000000, 0.000000000000000000, 1.000000000000000000 ) ) ;
#6381=ORIENTED_EDGE ( 'NONE', *, *, #5655, .F. ) ;
#6382=VERTEX_POINT ( 'NONE', #14221 ) ;
#6387=AXIS2_PLACEMENT_3D ( 'NONE', #1703, #7302, #6206 ) ;
#6390=ORIENTED_EDGE ( 'NONE', *, *, #8135, .T. ) ;
#6403=CARTESIAN_POINT ( 'NONE',  ( 145.1678582058265192, 408.6511750828049117, -210.0000000000000000 ) ) ;
#6406=CARTESIAN_POINT ( 'NONE',  ( 144.7991633467111683, 386.6211705227183870, -190.0000000000000000 ) ) ;
#6410=AXIS2_PLACEMENT_3D ( 'NONE', #6675, #2292, #5707 ) ;
#6412=DIRECTION ( 'NONE',  ( -0.000000000000000000, -0.000000000000000000, 1.000000000000000000 ) ) ;
#6417=DIRECTION ( 'NONE',  ( 1.000000000000000000, 0.000000000000000000, 0.000000000000000000 ) ) ;
#6422=ORIENTED_EDGE ( 'NONE', *, *, #11803, .T. ) ;
#6424=ORIENTED_EDGE ( 'NONE', *, *, #9772, .F. ) ;
#6431=CARTESIAN_POINT ( 'NONE',  ( 635.0000000000000000, 160.0000000000000284, 210.0000119999999981 ) ) ;
#6432=EDGE_CURVE ( 'NONE', #7052, #13396, #7952, .T. ) ;
#6434=PLANE ( 'NONE',  #12412 ) ;
#6435=CARTESIAN_POINT ( 'NONE',  ( 590.0000000000000000, 212.5596934910894333, 210.0000000000000000 ) ) ;
#6438=DIRECTION ( 'NONE',  ( -1.000000000000000000, 0.000000000000000000, 0.000000000000000000 ) ) ;
#6447=DIRECTION ( 'NONE',  ( -0.000000000000000000, -0.000000000000000000, 1.000000000000000000 ) ) ;
#6465=ORIENTED_EDGE ( 'NONE', *, *, #8542, .F. ) ;
#6469=CARTESIAN_POINT ( 'NONE',  ( 627.6952049249875927, 161.9631091326946830, 210.0000119999999981 ) ) ;
#6470=DIRECTION ( 'NONE',  ( -1.000000000000000000, 0.000000000000000000, 0.000000000000000000 ) ) ;
#6478=ADVANCED_FACE ( 'NONE', ( #8757 ), #14443, .F. ) ;
#6493=VERTEX_POINT ( 'NONE', #11987 ) ;
#6495=DIRECTION ( 'NONE',  ( 0.9578262852211513190, -0.2873478855663453846, 0.000000000000000000 ) ) ;
#6497=DIRECTION ( 'NONE',  ( -0.000000000000000000, -0.000000000000000000, 1.000000000000000000 ) ) ;
#6515=EDGE_LOOP ( 'NONE', ( #2478, #6465 ) ) ;
#6518=CARTESIAN_POINT ( 'NONE',  ( 610.0000000000000000, -9.999999999999941380, 210.0000000000000000 ) ) ;
#6535=CYLINDRICAL_SURFACE ( 'NONE', #5268, 2.649999999999985700 ) ;
#6546=EDGE_LOOP ( 'NONE', ( #7571, #7373, #1685, #3913 ) ) ;
#6547=DIRECTION ( 'NONE',  ( 0.000000000000000000, -1.000000000000000000, 0.000000000000000000 ) ) ;
#6552=DIRECTION ( 'NONE',  ( 0.000000000000000000, 0.000000000000000000, 1.000000000000000000 ) ) ;
#6556=VERTEX_POINT ( 'NONE', #79 ) ;
#6561=ADVANCED_FACE ( 'NONE', ( #990 ), #9105, .F. ) ;
#6563=VECTOR ( 'NONE', #14122, 1000.000000000000000 ) ;
#6565=DIRECTION ( 'NONE',  ( -0.000000000000000000, -0.000000000000000000, -1.000000000000000000 ) ) ;
#6567=CYLINDRICAL_SURFACE ( 'NONE', #4841, 7.500000000000062172 ) ;
#6573=EDGE_CURVE ( 'NONE', #13114, #6358, #13145, .T. ) ;
#6584=ORIENTED_EDGE ( 'NONE', *, *, #12332, .T. ) ;
#6588=PLANE ( 'NONE',  #5846 ) ;
#6606=CARTESIAN_POINT ( 'NONE',  ( 610.0000000000000000, 227.4403065089105951, -210.0000000000000000 ) ) ;
#6607=PLANE ( 'NONE',  #12687 ) ;
#6615=ORIENTED_EDGE ( 'NONE', *, *, #10660, .F. ) ;
#6616=DIRECTION ( 'NONE',  ( 0.000000000000000000, 1.000000000000000000, 0.000000000000000000 ) ) ;
#6617=AXIS2_PLACEMENT_3D ( 'NONE', #10737, #608, #7266 ) ;
#6635=ORIENTED_EDGE ( 'NONE', *, *, #10216, .F. ) ;
#6641=LINE ( 'NONE', #5378, #3778 ) ;
#6645=EDGE_CURVE ( 'NONE', #7999, #11993, #1126, .T. ) ;
#6651=LINE ( 'NONE', #12318, #11284 ) ;
#6668=ORIENTED_EDGE ( 'NONE', *, *, #9191, .F. ) ;
#6675=CARTESIAN_POINT ( 'NONE',  ( 635.0000000000000000, 160.0000000000000284, -190.0000000000000000 ) ) ;
#6682=FACE_OUTER_BOUND ( 'NONE', #5312, .T. ) ;
#6691=PLANE ( 'NONE',  #10393 ) ;
#6692=EDGE_CURVE ( 'NONE', #9303, #14092, #9487, .T. ) ;
#6694=ADVANCED_FACE ( 'NONE', ( #5853 ), #12722, .F. ) ;
#6698=DIRECTION ( 'NONE',  ( -0.000000000000000000, -0.000000000000000000, -1.000000000000000000 ) ) ;
#6707=DIRECTION ( 'NONE',  ( -0.2873478855663454401, -0.9578262852211514300, 0.000000000000000000 ) ) ;
#6712=DIRECTION ( 'NONE',  ( 0.2873478855663468279, 0.9578262852211509859, 0.000000000000000000 ) ) ;
#6726=EDGE_CURVE ( 'NONE', #13901, #2635, #9403, .T. ) ;
#6733=ORIENTED_EDGE ( 'NONE', *, *, #9883, .T. ) ;
#6743=CARTESIAN_POINT ( 'NONE',  ( 642.5000000000001137, 160.0000000000000284, 210.0000059999999849 ) ) ;
#6745=DIRECTION ( 'NONE',  ( 1.000000000000000000, 0.000000000000000000, 0.000000000000000000 ) ) ;
#6752=EDGE_CURVE ( 'NONE', #10194, #8820, #7256, .T. ) ;
#6753=ORIENTED_EDGE ( 'NONE', *, *, #10068, .T. ) ;
#6755=LINE ( 'NONE', #8897, #9938 ) ;
#6758=DIRECTION ( 'NONE',  ( 1.000000000000000000, 0.000000000000000000, 0.000000000000000000 ) ) ;
#6775=DIRECTION ( 'NONE',  ( -0.9578262852211517631, 0.2873478855663438858, 0.000000000000000000 ) ) ;
#6790=CARTESIAN_POINT ( 'NONE',  ( 164.3243839102495656, 402.9042173714779551, 210.0000000000000000 ) ) ;
#6792=EDGE_CURVE ( 'NONE', #10044, #902, #4838, .T. ) ;
#6798=VERTEX_POINT ( 'NONE', #9556 ) ;
#6803=VERTEX_POINT ( 'NONE', #14056 ) ;
#6820=LINE ( 'NONE', #80, #285 ) ;
#6831=CARTESIAN_POINT ( 'NONE',  ( 590.0000000000000000, -9.999999999999941380, -210.0020000000000095 ) ) ;
#6833=EDGE_LOOP ( 'NONE', ( #12122, #11226, #6026, #13999 ) ) ;
#6835=DIRECTION ( 'NONE',  ( 1.000000000000000000, 0.000000000000000000, 0.000000000000000000 ) ) ;
#6840=VECTOR ( 'NONE', #13101, 1000.000000000000000 ) ;
#6842=STYLED_ITEM ( 'NONE', ( #4273 ), #3907 ) ;
#6844=PRODUCT_DEFINITION ( 'UNKNOWN', '', #13028, #14471 ) ;
#6845=ORIENTED_EDGE ( 'NONE', *, *, #1000, .F. ) ;
#6847=VECTOR ( 'NONE', #6280, 1000.000000000000000 ) ;
#6851=CARTESIAN_POINT ( 'NONE',  ( 634.0059381729986399, 167.5000994061732911, -210.0000000000000000 ) ) ;
#6866=ORIENTED_EDGE ( 'NONE', *, *, #397, .T. ) ;
#6871=CIRCLE ( 'NONE', #1447, 5.249999999999976907 ) ;
#6878=CARTESIAN_POINT ( 'NONE',  ( 448.9584422793565750, 264.0194060144110608, -210.0000000000000000 ) ) ;
#6885=CARTESIAN_POINT ( 'NONE',  ( 627.6952049249875927, 158.0368908673054591, 210.0000120000000265 ) ) ;
#6892=ORIENTED_EDGE ( 'NONE', *, *, #1000, .T. ) ;
#6896=DIRECTION ( 'NONE',  ( -0.000000000000000000, 1.000000000000000000, 0.000000000000000000 ) ) ;
#6906=ORIENTED_EDGE ( 'NONE', *, *, #5170, .F. ) ;
#6911=DIRECTION ( 'NONE',  ( -1.000000000000000000, -0.000000000000000000, -0.000000000000000000 ) ) ;
#6927=DIRECTION ( 'NONE',  ( -0.2873478855663453846, -0.9578262852211513190, 0.000000000000000000 ) ) ;
#6930=CARTESIAN_POINT ( 'NONE',  ( 448.9584422793565750, 264.0194060144110608, 187.0000000000000000 ) ) ;
#6931=EDGE_LOOP ( 'NONE', ( #11681, #3335, #3058, #12599 ) ) ;
#6932=CARTESIAN_POINT ( 'NONE',  ( 145.1678582058265192, 408.6511750828049117, -210.0000000000000000 ) ) ;
#6941=DIRECTION ( 'NONE',  ( -1.000000000000000000, 0.000000000000000000, 0.000000000000000000 ) ) ;
#6942=ADVANCED_FACE ( 'NONE', ( #5895 ), #4876, .F. ) ;
#6947=ADVANCED_FACE ( 'NONE', ( #338 ), #13303, .F. ) ;
#6953=ORIENTED_EDGE ( 'NONE', *, *, #12311, .T. ) ;
#6954=ORIENTED_EDGE ( 'NONE', *, *, #9691, .T. ) ;
#6967=DIRECTION ( 'NONE',  ( -0.000000000000000000, -0.000000000000000000, 1.000000000000000000 ) ) ;
#6971=ORIENTED_EDGE ( 'NONE', *, *, #6645, .T. ) ;
#6973=CARTESIAN_POINT ( 'NONE',  ( 112.9652219749295341, 376.5507399164317803, -210.0000000000000000 ) ) ;
#6976=ORIENTED_EDGE ( 'NONE', *, *, #11248, .T. ) ;
#6978=PLANE ( 'NONE',  #8009 ) ;
#6981=DIRECTION ( 'NONE',  ( -0.000000000000000000, 0.000000000000000000, -1.000000000000000000 ) ) ;
#6985=LINE ( 'NONE', #2337, #1414 ) ;
#6992=FACE_OUTER_BOUND ( 'NONE', #6994, .T. ) ;
#6994=EDGE_LOOP ( 'NONE', ( #5589, #396, #6866, #2359 ) ) ;
#6996=CARTESIAN_POINT ( 'NONE',  ( 10.00000000000000000, -10.00000000000000000, -210.0020000000000095 ) ) ;
#7008=DIRECTION ( 'NONE',  ( 0.000000000000000000, 0.000000000000000000, -1.000000000000000000 ) ) ;
#7010=LINE ( 'NONE', #10267, #11137 ) ;
#7025=CARTESIAN_POINT ( 'NONE',  ( -10.00000000000000000, 0.000000000000000000, 210.0000000000000000 ) ) ;
#7030=ORIENTED_EDGE ( 'NONE', *, *, #10167, .T. ) ;
#7038=FACE_OUTER_BOUND ( 'NONE', #11795, .T. ) ;
#7052=VERTEX_POINT ( 'NONE', #8041 ) ;
#7065=ORIENTED_EDGE ( 'NONE', *, *, #10530, .T. ) ;
#7070=CYLINDRICAL_SURFACE ( 'NONE', #5653, 2.649999999999985700 ) ;
#7074=CARTESIAN_POINT ( 'NONE',  ( 610.0000000000000000, 145.0000000000000568, -210.0000000000000000 ) ) ;
#7075=EDGE_LOOP ( 'NONE', ( #7518, #9493, #8924, #4111 ) ) ;
#7086=CARTESIAN_POINT ( 'NONE',  ( 142.4540310085880606, 355.9707293956415697, 187.0000000000000000 ) ) ;
#7095=PLANE ( 'NONE',  #14575 ) ;
#7099=VERTEX_POINT ( 'NONE', #12837 ) ;
#7106=DIRECTION ( 'NONE',  ( 0.000000000000000000, 0.000000000000000000, -1.000000000000000000 ) ) ;
#7113=VECTOR ( 'NONE', #7709, 1000.000000000000000 ) ;
#7133=FACE_OUTER_BOUND ( 'NONE', #2257, .T. ) ;
#7139=EDGE_CURVE ( 'NONE', #9301, #4023, #854, .T. ) ;
#7140=FACE_OUTER_BOUND ( 'NONE', #9708, .T. ) ;
#7142=EDGE_CURVE ( 'NONE', #10448, #2847, #12154, .T. ) ;
#7157=ORIENTED_EDGE ( 'NONE', *, *, #2864, .T. ) ;
#7160=ORIENTED_EDGE ( 'NONE', *, *, #2207, .F. ) ;
#7168=DIRECTION ( 'NONE',  ( 1.000000000000000000, 0.000000000000000000, 0.000000000000000000 ) ) ;
#7178=CARTESIAN_POINT ( 'NONE',  ( -10.00000000000000000, 10.00000000000000178, -190.0000000000000000 ) ) ;
#7181=VERTEX_POINT ( 'NONE', #1152 ) ;
#7193=EDGE_LOOP ( 'NONE', ( #13840, #11052, #6953, #8078 ) ) ;
#7203=FACE_OUTER_BOUND ( 'NONE', #3715, .T. ) ;
#7213=CARTESIAN_POINT ( 'NONE',  ( 650.0000000000000000, 175.0000000000000568, -210.0000000000000000 ) ) ;
#7218=FACE_OUTER_BOUND ( 'NONE', #1037, .T. ) ;
#7221=ORIENTED_EDGE ( 'NONE', *, *, #7, .T. ) ;
#7228=CARTESIAN_POINT ( 'NONE',  ( 107.2182642636026202, 357.3942142120087055, 190.0000000000000000 ) ) ;
#7231=CARTESIAN_POINT ( 'NONE',  ( 470.8287951810180516, 310.9528939902474463, 210.0000000000000000 ) ) ;
#7236=FACE_BOUND ( 'NONE', #9929, .T. ) ;
#7244=DIRECTION ( 'NONE',  ( 0.000000000000000000, 1.000000000000000000, 0.000000000000000000 ) ) ;
#7246=EDGE_CURVE ( 'NONE', #6340, #6556, #12441, .T. ) ;
#7256=LINE ( 'NONE', #11744, #8666 ) ;
#7257=LINE ( 'NONE', #1507, #1260 ) ;
#7261=EDGE_LOOP ( 'NONE', ( #2103, #2578 ) ) ;
#7263=CYLINDRICAL_SURFACE ( 'NONE', #2382, 2.649999999999985700 ) ;
#7266=DIRECTION ( 'NONE',  ( 1.000000000000000000, 0.000000000000000000, 0.000000000000000000 ) ) ;
#7268=LINE ( 'NONE', #8225, #5368 ) ;
#7280=CARTESIAN_POINT ( 'NONE',  ( 0.000000000000000000, 0.000000000000000000, -190.0000000000000000 ) ) ;
#7290=( LENGTH_UNIT ( ) NAMED_UNIT ( * ) SI_UNIT ( .MILLI., .METRE. ) );
#7292=ORIENTED_EDGE ( 'NONE', *, *, #6301, .F. ) ;
#7302=DIRECTION ( 'NONE',  ( -0.2873478855663454401, -0.9578262852211514300, 0.000000000000000000 ) ) ;
#7305=LINE ( 'NONE', #7231, #10625 ) ;
#7313=ADVANCED_FACE ( 'NONE', ( #1306 ), #5803, .T. ) ;
#7314=VECTOR ( 'NONE', #13091, 1000.000000000000000 ) ;
#7315=EDGE_LOOP ( 'NONE', ( #11033, #9022, #8987, #12342 ) ) ;
#7325=ORIENTED_EDGE ( 'NONE', *, *, #12653, .F. ) ;
#7336=ORIENTED_EDGE ( 'NONE', *, *, #11248, .F. ) ;
#7345=CARTESIAN_POINT ( 'NONE',  ( 610.0000000000000000, 0.000000000000000000, 190.0000000000000000 ) ) ;
#7346=CARTESIAN_POINT ( 'NONE',  ( 451.6722694765949768, 316.6998517015743460, 210.0000000000000000 ) ) ;
#7347=EDGE_LOOP ( 'NONE', ( #13768, #2013 ) ) ;
#7351=CARTESIAN_POINT ( 'NONE',  ( -10.00000000000000000, -10.00000000000000000, -210.0000000000000000 ) ) ;
#7355=ORIENTED_EDGE ( 'NONE', *, *, #11337, .F. ) ;
#7366=( GEOMETRIC_REPRESENTATION_CONTEXT ( 3 ) GLOBAL_UNCERTAINTY_ASSIGNED_CONTEXT ( ( #3561 ) ) GLOBAL_UNIT_ASSIGNED_CONTEXT ( ( #1076, #5874, #10236 ) ) REPRESENTATION_CONTEXT ( 'NONE', 'WORKASPACE' ) );
#7369=ADVANCED_FACE ( 'NONE', ( #11697, #8235, #10603, #5145, #10746, #7140 ), #11633, .F. ) ;
#7373=ORIENTED_EDGE ( 'NONE', *, *, #6752, .F. ) ;
#7385=DIRECTION ( 'NONE',  ( -1.000000000000000000, 0.000000000000000000, 0.000000000000000000 ) ) ;
#7394=DIRECTION ( 'NONE',  ( 0.9578262852211517631, -0.2873478855663438858, 0.000000000000000000 ) ) ;
#7397=EDGE_CURVE ( 'NONE', #14524, #3289, #1591, .T. ) ;
#7402=LINE ( 'NONE', #13084, #2607 ) ;
#7413=CARTESIAN_POINT ( 'NONE',  ( 610.0000000000000000, 227.4403065089105951, -190.0000000000000000 ) ) ;
#7418=CARTESIAN_POINT ( 'NONE',  ( 139.8040310085880833, 355.9707293956415697, 187.0000000000000000 ) ) ;
#7424=DIRECTION ( 'NONE',  ( -1.000000000000000000, -0.000000000000000000, -0.000000000000000000 ) ) ;
#7447=CYLINDRICAL_SURFACE ( 'NONE', #12468, 5.249999999999976907 ) ;
#7448=EDGE_CURVE ( 'NONE', #3152, #10585, #5227, .T. ) ;
#7450=DIRECTION ( 'NONE',  ( 1.000000000000000000, 0.000000000000000000, 0.000000000000000000 ) ) ;
#7457=DIRECTION ( 'NONE',  ( 0.000000000000000000, 1.000000000000000000, 0.000000000000000000 ) ) ;
#7460=FACE_OUTER_BOUND ( 'NONE', #13112, .T. ) ;
#7469=CARTESIAN_POINT ( 'NONE',  ( 10.00000000000000000, -9.999999999999998224, -190.0000000000000000 ) ) ;
#7470=DIRECTION ( 'NONE',  ( -0.000000000000000000, -0.000000000000000000, -1.000000000000000000 ) ) ;
#7481=ORIENTED_EDGE ( 'NONE', *, *, #13985, .F. ) ;
#7486=VECTOR ( 'NONE', #4668, 1000.000000000000000 ) ;
#7489=CARTESIAN_POINT ( 'NONE',  ( 634.0182522957533138, 167.5000000000000568, 210.0000119999999981 ) ) ;
#7501=CARTESIAN_POINT ( 'NONE',  ( 590.0000000000000000, -9.999999999999941380, 190.0000000000000000 ) ) ;
#7502=LINE ( 'NONE', #1896, #9230 ) ;
#7506=VERTEX_POINT ( 'NONE', #11183 ) ;
#7510=ADVANCED_FACE ( 'NONE', ( #2240 ), #1356, .T. ) ;
#7513=EDGE_CURVE ( 'NONE', #6803, #542, #10224, .T. ) ;
#7517=VECTOR ( 'NONE', #2858, 1000.000000000000000 ) ;
#7518=ORIENTED_EDGE ( 'NONE', *, *, #9547, .F. ) ;
#7524=FACE_OUTER_BOUND ( 'NONE', #50, .T. ) ;
#7525=VECTOR ( 'NONE', #1402, 1000.000000000000000 ) ;
#7526=VECTOR ( 'NONE', #12517, 1000.000000000000000 ) ;
#7530=EDGE_LOOP ( 'NONE', ( #4334, #7065, #11157, #9568 ) ) ;
#7532=LINE ( 'NONE', #6435, #8938 ) ;
#7541=EDGE_CURVE ( 'NONE', #11118, #1544, #3302, .T. ) ;
#7549=CARTESIAN_POINT ( 'NONE',  ( 440.1783540539412343, 278.3868002927283101, 190.0000000000000000 ) ) ;
#7553=( GEOMETRIC_REPRESENTATION_CONTEXT ( 3 ) GLOBAL_UNCERTAINTY_ASSIGNED_CONTEXT ( ( #7847 ) ) GLOBAL_UNIT_ASSIGNED_CONTEXT ( ( #7290, #14086, #634 ) ) REPRESENTATION_CONTEXT ( 'NONE', 'WORKASPACE' ) );
#7556=DIRECTION ( 'NONE',  ( -1.000000000000000000, 0.000000000000000000, 0.000000000000000000 ) ) ;
#7566=VECTOR ( 'NONE', #14465, 1000.000000000000114 ) ;
#7571=ORIENTED_EDGE ( 'NONE', *, *, #1335, .F. ) ;
#7580=CARTESIAN_POINT ( 'NONE',  ( 635.0000000000000000, 160.0000000000000284, 210.0000119999999981 ) ) ;
#7581=EDGE_LOOP ( 'NONE', ( #9452, #11538, #4693, #8624 ) ) ;
#7583=EDGE_LOOP ( 'NONE', ( #9968, #7600, #11232, #3697 ) ) ;
#7585=VECTOR ( 'NONE', #10183, 1000.000000000000114 ) ;
#7594=FILL_AREA_STYLE_COLOUR ( '', #13210 ) ;
#7597=ADVANCED_FACE ( 'NONE', ( #7872 ), #12421, .F. ) ;
#7598=DIRECTION ( 'NONE',  ( -0.2873478855663453846, -0.9578262852211513190, -0.000000000000000000 ) ) ;
#7600=ORIENTED_EDGE ( 'NONE', *, *, #7513, .F. ) ;
#7602=ORIENTED_EDGE ( 'NONE', *, *, #4135, .T. ) ;
#7613=LINE ( 'NONE', #13075, #9124 ) ;
#7622=EDGE_LOOP ( 'NONE', ( #7336, #4914, #9536, #657 ) ) ;
#7637=ORIENTED_EDGE ( 'NONE', *, *, #10461, .F. ) ;
#7643=ADVANCED_FACE ( 'NONE', ( #7038 ), #3814, .T. ) ;
#7649=CARTESIAN_POINT ( 'NONE',  ( 627.5000000000000000, 160.0000000000000284, 210.0000059999999849 ) ) ;
#7653=LINE ( 'NONE', #8826, #13046 ) ;
#7665=DIRECTION ( 'NONE',  ( -0.000000000000000000, -0.000000000000000000, 1.000000000000000000 ) ) ;
#7676=CARTESIAN_POINT ( 'NONE',  ( 630.3995367089856927, 153.9937209916067786, -210.0000000000000000 ) ) ;
#7678=VECTOR ( 'NONE', #11589, 1000.000000000000114 ) ;
#7700=ORIENTED_EDGE ( 'NONE', *, *, #7139, .T. ) ;
#7702=EDGE_LOOP ( 'NONE', ( #3286, #11197, #4720, #6668 ) ) ;
#7709=DIRECTION ( 'NONE',  ( 0.000000000000000000, -1.000000000000000000, 0.000000000000000000 ) ) ;
#7710=LINE ( 'NONE', #5505, #5194 ) ;
#7722=VECTOR ( 'NONE', #13754, 1000.000000000000000 ) ;
#7725=DIRECTION ( 'NONE',  ( 1.000000000000000000, 0.000000000000000000, 0.000000000000000000 ) ) ;
#7726=CARTESIAN_POINT ( 'NONE',  ( 610.0000000000000000, 0.000000000000000000, 210.0000000000000000 ) ) ;
#7727=ORIENTED_EDGE ( 'NONE', *, *, #3637, .F. ) ;
#7728=FACE_OUTER_BOUND ( 'NONE', #675, .T. ) ;
#7739=CIRCLE ( 'NONE', #13392, 2.649999999999985700 ) ;
#7741=DIRECTION ( 'NONE',  ( -1.000000000000000000, 0.000000000000000000, 0.000000000000000000 ) ) ;
#7742=VECTOR ( 'NONE', #14486, 1000.000000000000000 ) ;
#7746=DIRECTION ( 'NONE',  ( -0.000000000000000000, -0.000000000000000000, -1.000000000000000000 ) ) ;
#7750=ORIENTED_EDGE ( 'NONE', *, *, #1954, .F. ) ;
#7758=ORIENTED_EDGE ( 'NONE', *, *, #2161, .F. ) ;
#7765=VERTEX_POINT ( 'NONE', #14343 ) ;
#7796=ORIENTED_EDGE ( 'NONE', *, *, #970, .F. ) ;
#7805=DIRECTION ( 'NONE',  ( -0.2873478855663453846, -0.9578262852211513190, -0.000000000000000000 ) ) ;
#7806=EDGE_LOOP ( 'NONE', ( #2558, #5418, #9577, #7637 ) ) ;
#7811=DIRECTION ( 'NONE',  ( 1.000000000000000000, 9.498873539028489960E-17, 0.000000000000000000 ) ) ;
#7813=ORIENTED_EDGE ( 'NONE', *, *, #10954, .F. ) ;
#7819=DIRECTION ( 'NONE',  ( -0.000000000000000000, -0.000000000000000000, -1.000000000000000000 ) ) ;
#7820=DIRECTION ( 'NONE',  ( -0.000000000000000000, -0.000000000000000000, -1.000000000000000000 ) ) ;
#7831=EDGE_LOOP ( 'NONE', ( #9062, #5483 ) ) ;
#7840=VECTOR ( 'NONE', #8246, 1000.000000000000000 ) ;
#7842=CARTESIAN_POINT ( 'NONE',  ( 148.9991633467111569, 386.6211705227183870, -190.0000000000000000 ) ) ;
#7843=CARTESIAN_POINT ( 'NONE',  ( 650.0000000000000000, 175.0000000000000568, 210.0000000000000000 ) ) ;
#7847=UNCERTAINTY_MEASURE_WITH_UNIT (LENGTH_MEASURE( 1.000000000000000082E-05 ), #7290, 'distance_accuracy_value', 'NONE');
#7856=ORIENTED_EDGE ( 'NONE', *, *, #1784, .F. ) ;
#7872=FACE_OUTER_BOUND ( 'NONE', #12060, .T. ) ;
#7885=CARTESIAN_POINT ( 'NONE',  ( 650.0000000000000000, 175.0000000000000568, 190.0000000000000000 ) ) ;
#7886=VERTEX_POINT ( 'NONE', #7917 ) ;
#7888=EDGE_LOOP ( 'NONE', ( #5005, #5049, #8517, #9077 ) ) ;
#7889=CARTESIAN_POINT ( 'NONE',  ( 9.498873539028489220E-16, -10.00000000000000000, 190.0000000000000000 ) ) ;
#7890=CARTESIAN_POINT ( 'NONE',  ( 139.8040310085880833, 355.9707293956415697, -210.0000000000000000 ) ) ;
#7903=EDGE_LOOP ( 'NONE', ( #1751, #3084, #8716, #1746 ) ) ;
#7908=DIRECTION ( 'NONE',  ( 0.000000000000000000, 1.000000000000000000, 0.000000000000000000 ) ) ;
#7910=DIRECTION ( 'NONE',  ( -0.9578262852211513190, 0.2873478855663453846, 0.000000000000000000 ) ) ;
#7917=CARTESIAN_POINT ( 'NONE',  ( 640.2500000000000000, 160.0000000000000284, 190.0000000000000284 ) ) ;
#7918=ORIENTED_EDGE ( 'NONE', *, *, #7246, .T. ) ;
#7919=ORIENTED_EDGE ( 'NONE', *, *, #7397, .F. ) ;
#7922=EDGE_CURVE ( 'NONE', #2271, #11363, #5704, .T. ) ;
#7926=ORIENTED_EDGE ( 'NONE', *, *, #14145, .T. ) ;
#7927=CARTESIAN_POINT ( 'NONE',  ( 148.9991633467111569, 386.6211705227183870, 190.0000000000000000 ) ) ;
#7928=DIRECTION ( 'NONE',  ( -0.000000000000000000, -0.000000000000000000, 1.000000000000000000 ) ) ;
#7934=EDGE_LOOP ( 'NONE', ( #857, #385 ) ) ;
#7941=CARTESIAN_POINT ( 'NONE',  ( 137.1540310085880776, 355.9707293956415697, 190.0000000000000000 ) ) ;
#7944=VERTEX_POINT ( 'NONE', #9094 ) ;
#7952=CIRCLE ( 'NONE', #11256, 2.649999999999985700 ) ;
#7956=EDGE_CURVE ( 'NONE', #6358, #13114, #10379, .T. ) ;
#7965=AXIS2_PLACEMENT_3D ( 'NONE', #7346, #10674, #6091 ) ;
#7976=ORIENTED_EDGE ( 'NONE', *, *, #2986, .F. ) ;
#7978=CARTESIAN_POINT ( 'NONE',  ( 133.6739427831727198, 370.3381236739588758, -210.0000000000000000 ) ) ;
#7980=DIRECTION ( 'NONE',  ( 1.000000000000000000, 0.000000000000000000, 0.000000000000000000 ) ) ;
#7987=ADVANCED_FACE ( 'NONE', ( #13456 ), #3352, .T. ) ;
#7995=LINE ( 'NONE', #8073, #10085 ) ;
#7999=VERTEX_POINT ( 'NONE', #12402 ) ;
#8009=AXIS2_PLACEMENT_3D ( 'NONE', #12817, #5872, #10378 ) ;
#8010=FACE_OUTER_BOUND ( 'NONE', #359, .T. ) ;
#8012=AXIS2_PLACEMENT_3D ( 'NONE', #7842, #11373, #6941 ) ;
#8014=CARTESIAN_POINT ( 'NONE',  ( 650.0000000000000000, 145.0000000000000568, 190.0000000000000000 ) ) ;
#8021=AXIS2_PLACEMENT_3D ( 'NONE', #10157, #12430, #10229 ) ;
#8028=CARTESIAN_POINT ( 'NONE',  ( 642.5000000000001137, 160.0000000000000284, -210.0000059999999849 ) ) ;
#8031=ADVANCED_FACE ( 'NONE', ( #5048 ), #8124, .F. ) ;
#8034=EDGE_CURVE ( 'NONE', #8972, #5634, #291, .T. ) ;
#8037=VECTOR ( 'NONE', #9068, 1000.000000000000000 ) ;
#8041=CARTESIAN_POINT ( 'NONE',  ( 137.1540310085880776, 355.9707293956415697, -210.0000000000000000 ) ) ;
#8048=EDGE_LOOP ( 'NONE', ( #4457, #5691, #7481, #1129 ) ) ;
#8052=AXIS2_PLACEMENT_3D ( 'NONE', #3583, #8881, #8071 ) ;
#8053=DIRECTION ( 'NONE',  ( 0.9578262852211513190, -0.2873478855663453846, 0.000000000000000000 ) ) ;
#8054=LINE ( 'NONE', #1185, #13852 ) ;
#8059=VECTOR ( 'NONE', #1251, 1000.000000000000114 ) ;
#8065=EDGE_CURVE ( 'NONE', #12523, #5769, #8743, .T. ) ;
#8067=CARTESIAN_POINT ( 'NONE',  ( 9.498873539028489220E-16, -10.00000000000000000, -190.0000000000000000 ) ) ;
#8068=CARTESIAN_POINT ( 'NONE',  ( 635.0000000000000000, 160.0000000000000284, -210.0000000000000000 ) ) ;
#8069=ORIENTED_EDGE ( 'NONE', *, *, #14083, .F. ) ;
#8071=DIRECTION ( 'NONE',  ( 1.000000000000000000, 0.000000000000000000, 0.000000000000000000 ) ) ;
#8073=CARTESIAN_POINT ( 'NONE',  ( -10.00000000000000000, 413.4403065089105667, 210.0000000000000000 ) ) ;
#8078=ORIENTED_EDGE ( 'NONE', *, *, #10260, .T. ) ;
#8079=EDGE_LOOP ( 'NONE', ( #14080, #1394, #1031, #565 ) ) ;
#8087=DIRECTION ( 'NONE',  ( 0.000000000000000000, 0.000000000000000000, 1.000000000000000000 ) ) ;
#8089=VECTOR ( 'NONE', #9035, 1000.000000000000114 ) ;
#8099=EDGE_CURVE ( 'NONE', #3368, #7099, #13751, .T. ) ;
#8111=ORIENTED_EDGE ( 'NONE', *, *, #12332, .F. ) ;
#8116=LINE ( 'NONE', #7086, #7525 ) ;
#8121=DIRECTION ( 'NONE',  ( -0.000000000000000000, -0.000000000000000000, -1.000000000000000000 ) ) ;
#8124=PLANE ( 'NONE',  #9922 ) ;
#8127=CARTESIAN_POINT ( 'NONE',  ( 635.9817477042469136, 152.4999999999999716, 210.0000119999999981 ) ) ;
#8135=EDGE_CURVE ( 'NONE', #12947, #9303, #5261, .T. ) ;
#8139=VERTEX_POINT ( 'NONE', #6356 ) ;
#8147=LINE ( 'NONE', #12656, #4770 ) ;
#8148=ADVANCED_FACE ( 'NONE', ( #14189 ), #8497, .F. ) ;
#8150=ADVANCED_FACE ( 'NONE', ( #9823 ), #6276, .F. ) ;
#8159=CARTESIAN_POINT ( 'NONE',  ( 610.0000000000000000, 175.0000000000000568, -190.0000000000000000 ) ) ;
#8165=EDGE_CURVE ( 'NONE', #9542, #13868, #3036, .T. ) ;
#8169=DIRECTION ( 'NONE',  ( -0.000000000000000000, -0.000000000000000000, -1.000000000000000000 ) ) ;
#8174=EDGE_CURVE ( 'NONE', #5554, #11494, #4266, .T. ) ;
#8187=ORIENTED_EDGE ( 'NONE', *, *, #281, .F. ) ;
#8211=CARTESIAN_POINT ( 'NONE',  ( 610.0000000000000000, 145.0000000000000568, 210.0000000000000000 ) ) ;
#8218=EDGE_LOOP ( 'NONE', ( #10886, #928, #10540, #8740 ) ) ;
#8225=CARTESIAN_POINT ( 'NONE',  ( 145.1678582058265476, 408.6511750828048548, -190.0000000000000000 ) ) ;
#8229=DIRECTION ( 'NONE',  ( 0.000000000000000000, -1.000000000000000000, 0.000000000000000000 ) ) ;
#8235=FACE_BOUND ( 'NONE', #4400, .T. ) ;
#8237=VECTOR ( 'NONE', #14295, 1000.000000000000000 ) ;
#8246=DIRECTION ( 'NONE',  ( 0.000000000000000000, 0.000000000000000000, -1.000000000000000000 ) ) ;
#8250=CARTESIAN_POINT ( 'NONE',  ( -10.00000000000000000, 0.000000000000000000, 190.0000000000000000 ) ) ;
#8251=ORIENTED_EDGE ( 'NONE', *, *, #12653, .T. ) ;
#8253=AXIS2_PLACEMENT_3D ( 'NONE', #2375, #4447, #7980 ) ;
#8257=CARTESIAN_POINT ( 'NONE',  ( 446.3084422793565409, 264.0194060144110608, 190.0000000000000000 ) ) ;
#8262=EDGE_CURVE ( 'NONE', #6382, #5721, #10934, .T. ) ;
#8270=EDGE_CURVE ( 'NONE', #10585, #8972, #13144, .T. ) ;
#8282=DIRECTION ( 'NONE',  ( 1.000000000000000000, 9.498873539028489960E-17, 0.000000000000000000 ) ) ;
#8286=VERTEX_POINT ( 'NONE', #3333 ) ;
#8288=DIRECTION ( 'NONE',  ( 0.000000000000000000, -1.000000000000000000, 0.000000000000000000 ) ) ;
#8290=DIRECTION ( 'NONE',  ( -0.2873478855663453846, -0.9578262852211513190, -0.000000000000000000 ) ) ;
#8293=DIRECTION ( 'NONE',  ( 1.000000000000000000, 0.000000000000000000, -0.000000000000000000 ) ) ;
#8300=DIRECTION ( 'NONE',  ( -0.000000000000000000, -0.000000000000000000, -1.000000000000000000 ) ) ;
#8328=LINE ( 'NONE', #12838, #5131 ) ;
#8335=DIRECTION ( 'NONE',  ( -1.000000000000000000, 0.000000000000000000, 0.000000000000000000 ) ) ;
#8346=CARTESIAN_POINT ( 'NONE',  ( 112.9652219749295341, 376.5507399164317803, -210.0000000000000000 ) ) ;
#8349=ORIENTED_EDGE ( 'NONE', *, *, #8165, .F. ) ;
#8350=DIRECTION ( 'NONE',  ( 1.000000000000000000, 0.000000000000000000, 0.000000000000000000 ) ) ;
#8363=CARTESIAN_POINT ( 'NONE',  ( 142.4540310085880606, 355.9707293956415697, 190.0000000000000000 ) ) ;
#8377=VERTEX_POINT ( 'NONE', #116 ) ;
#8386=FACE_BOUND ( 'NONE', #2402, .T. ) ;
#8402=PLANE ( 'NONE',  #6387 ) ;
#8405=CARTESIAN_POINT ( 'NONE',  ( 451.3035746174796827, 294.6698471414878782, -210.0000000000000000 ) ) ;
#8409=DIRECTION ( 'NONE',  ( -0.000000000000000000, -0.000000000000000000, 1.000000000000000000 ) ) ;
#8413=CARTESIAN_POINT ( 'NONE',  ( 635.0000000000000000, 160.0000000000000284, -190.0000000000000000 ) ) ;
#8415=ORIENTED_EDGE ( 'NONE', *, *, #322, .T. ) ;
#8430=ORIENTED_EDGE ( 'NONE', *, *, #1784, .T. ) ;
#8433=ORIENTED_EDGE ( 'NONE', *, *, #311, .F. ) ;
#8439=CARTESIAN_POINT ( 'NONE',  ( 610.0000000000000000, 175.0000000000000568, 190.0000000000000000 ) ) ;
#8441=ORIENTED_EDGE ( 'NONE', *, *, #5612, .T. ) ;
#8445=VECTOR ( 'NONE', #1158, 1000.000000000000000 ) ;
#8457=ORIENTED_EDGE ( 'NONE', *, *, #14251, .T. ) ;
#8460=VECTOR ( 'NONE', #8282, 1000.000000000000000 ) ;
#8471=ORIENTED_EDGE ( 'NONE', *, *, #12706, .F. ) ;
#8475=LINE ( 'NONE', #8250, #9845 ) ;
#8482=CYLINDRICAL_SURFACE ( 'NONE', #3280, 2.649999999999985700 ) ;
#8496=VECTOR ( 'NONE', #10589, 1000.000000000000114 ) ;
#8497=PLANE ( 'NONE',  #13693 ) ;
#8502=DIRECTION ( 'NONE',  ( -0.9578262852211513190, 0.2873478855663453846, 0.000000000000000000 ) ) ;
#8506=AXIS2_PLACEMENT_3D ( 'NONE', #1531, #1313, #1246 ) ;
#8511=DIRECTION ( 'NONE',  ( -1.000000000000000000, 0.000000000000000000, 0.000000000000000000 ) ) ;
#8517=ORIENTED_EDGE ( 'NONE', *, *, #8696, .T. ) ;
#8526=AXIS2_PLACEMENT_3D ( 'NONE', #2250, #8087, #4708 ) ;
#8528=CARTESIAN_POINT ( 'NONE',  ( 635.0000000000000000, 160.0000000000000284, -210.0000119999999981 ) ) ;
#8530=LINE ( 'NONE', #13106, #5889 ) ;
#8542=EDGE_CURVE ( 'NONE', #10517, #10228, #5218, .T. ) ;
#8558=EDGE_LOOP ( 'NONE', ( #10193, #11770, #2522, #4591 ) ) ;
#8569=FACE_OUTER_BOUND ( 'NONE', #1610, .T. ) ;
#8574=DIRECTION ( 'NONE',  ( -0.2873478855663454401, -0.9578262852211514300, 0.000000000000000000 ) ) ;
#8576=ORIENTED_EDGE ( 'NONE', *, *, #12240, .F. ) ;
#8592=ORIENTED_EDGE ( 'NONE', *, *, #10915, .T. ) ;
#8595=CARTESIAN_POINT ( 'NONE',  ( -10.00000000000000000, -10.00000000000000000, 210.0000000000000000 ) ) ;
#8598=ADVANCED_FACE ( 'NONE', ( #781 ), #6691, .F. ) ;
#8605=VERTEX_POINT ( 'NONE', #4335 ) ;
#8609=DIRECTION ( 'NONE',  ( 0.2873478855663453846, 0.9578262852211513190, 0.000000000000000000 ) ) ;
#8614=ORIENTED_EDGE ( 'NONE', *, *, #2130, .T. ) ;
#8621=EDGE_CURVE ( 'NONE', #3017, #9599, #915, .T. ) ;
#8624=ORIENTED_EDGE ( 'NONE', *, *, #12878, .T. ) ;
#8626=ORIENTED_EDGE ( 'NONE', *, *, #8174, .F. ) ;
#8636=DIRECTION ( 'NONE',  ( -0.9578262852211515410, 0.2873478855663446074, 0.000000000000000000 ) ) ;
#8639=CARTESIAN_POINT ( 'NONE',  ( 451.6722694765949768, 316.6998517015743460, 210.0000000000000000 ) ) ;
#8645=LINE ( 'NONE', #13149, #8725 ) ;
#8652=VECTOR ( 'NONE', #1841, 1000.000000000000000 ) ;
#8659=ORIENTED_EDGE ( 'NONE', *, *, #9883, .F. ) ;
#8666=VECTOR ( 'NONE', #5940, 1000.000000000000114 ) ;
#8668=ORIENTED_EDGE ( 'NONE', *, *, #11070, .F. ) ;
#8682=ADVANCED_FACE ( 'NONE', ( #3290 ), #4181, .F. ) ;
#8685=LINE ( 'NONE', #5020, #14413 ) ;
#8696=EDGE_CURVE ( 'NONE', #4375, #12665, #11117, .T. ) ;
#8705=AXIS2_PLACEMENT_3D ( 'NONE', #7843, #9261, #2061 ) ;
#8714=AXIS2_PLACEMENT_3D ( 'NONE', #254, #2479, #6981 ) ;
#8715=DIRECTION ( 'NONE',  ( -0.9578262852211513190, 0.2873478855663453846, 0.000000000000000000 ) ) ;
#8716=ORIENTED_EDGE ( 'NONE', *, *, #1425, .F. ) ;
#8725=VECTOR ( 'NONE', #1931, 1000.000000000000000 ) ;
#8728=VERTEX_POINT ( 'NONE', #6406 ) ;
#8739=ORIENTED_EDGE ( 'NONE', *, *, #14145, .F. ) ;
#8740=ORIENTED_EDGE ( 'NONE', *, *, #3135, .T. ) ;
#8742=DIRECTION ( 'NONE',  ( -0.2873478855663453846, -0.9578262852211513190, -0.000000000000000000 ) ) ;
#8743=CIRCLE ( 'NONE', #2116, 5.249999999999976907 ) ;
#8749=ORIENTED_EDGE ( 'NONE', *, *, #1326, .F. ) ;
#8757=FACE_OUTER_BOUND ( 'NONE', #7193, .T. ) ;
#8770=CARTESIAN_POINT ( 'NONE',  ( 145.1678582058265476, 408.6511750828048548, -190.0000000000000000 ) ) ;
#8777=EDGE_LOOP ( 'NONE', ( #8867, #5223 ) ) ;
#8781=ORIENTED_EDGE ( 'NONE', *, *, #13561, .F. ) ;
#8783=CARTESIAN_POINT ( 'NONE',  ( 650.0000000000000000, 175.0000000000000568, -210.0000000000000000 ) ) ;
#8790=VERTEX_POINT ( 'NONE', #10227 ) ;
#8805=VERTEX_POINT ( 'NONE', #85 ) ;
#8819=DIRECTION ( 'NONE',  ( 0.000000000000000000, -1.000000000000000000, 0.000000000000000000 ) ) ;
#8820=VERTEX_POINT ( 'NONE', #3598 ) ;
#8826=CARTESIAN_POINT ( 'NONE',  ( 650.0000000000000000, 145.0000000000000568, 210.0000000000000000 ) ) ;
#8838=DIRECTION ( 'NONE',  ( 0.000000000000000000, 0.000000000000000000, -1.000000000000000000 ) ) ;
#8841=ORIENTED_EDGE ( 'NONE', *, *, #10128, .F. ) ;
#8865=PLANE ( 'NONE',  #8705 ) ;
#8867=ORIENTED_EDGE ( 'NONE', *, *, #6080, .F. ) ;
#8868=DIRECTION ( 'NONE',  ( 0.000000000000000000, 1.000000000000000000, 0.000000000000000000 ) ) ;
#8876=EDGE_CURVE ( 'NONE', #1729, #197, #2920, .T. ) ;
#8881=DIRECTION ( 'NONE',  ( 0.000000000000000000, 0.000000000000000000, -1.000000000000000000 ) ) ;
#8885=CARTESIAN_POINT ( 'NONE',  ( -10.00000000000000000, 413.4403065089105667, -210.0000000000000000 ) ) ;
#8889=ORIENTED_EDGE ( 'NONE', *, *, #10418, .T. ) ;
#8891=EDGE_CURVE ( 'NONE', #8139, #7944, #9563, .T. ) ;
#8896=ADVANCED_FACE ( 'NONE', ( #4026 ), #7263, .F. ) ;
#8897=CARTESIAN_POINT ( 'NONE',  ( 137.1540310085880776, 355.9707293956415697, 187.0000000000000000 ) ) ;
#8900=DIRECTION ( 'NONE',  ( 0.000000000000000000, 0.000000000000000000, 1.000000000000000000 ) ) ;
#8901=DIRECTION ( 'NONE',  ( -1.000000000000000000, 0.000000000000000000, 0.000000000000000000 ) ) ;
#8915=LINE ( 'NONE', #8783, #919 ) ;
#8923=DIRECTION ( 'NONE',  ( -0.9578262852211508749, 0.2873478855663467724, 0.000000000000000000 ) ) ;
#8924=ORIENTED_EDGE ( 'NONE', *, *, #10915, .F. ) ;
#8930=EDGE_CURVE ( 'NONE', #1538, #8790, #6168, .T. ) ;
#8937=VECTOR ( 'NONE', #11135, 1000.000000000000000 ) ;
#8938=VECTOR ( 'NONE', #12026, 1000.000000000000000 ) ;
#8952=DIRECTION ( 'NONE',  ( -1.000000000000000000, 0.000000000000000000, 0.000000000000000000 ) ) ;
#8955=CARTESIAN_POINT ( 'NONE',  ( 440.1783540539411774, 278.3868002927282532, -210.0000000000000000 ) ) ;
#8967=VECTOR ( 'NONE', #3253, 1000.000000000000000 ) ;
#8972=VERTEX_POINT ( 'NONE', #6085 ) ;
#8984=CARTESIAN_POINT ( 'NONE',  ( 0.000000000000000000, 0.000000000000000000, -190.0000000000000000 ) ) ;
#8987=ORIENTED_EDGE ( 'NONE', *, *, #6073, .T. ) ;
#8999=VECTOR ( 'NONE', #4788, 1000.000000000000000 ) ;
#9004=ORIENTED_EDGE ( 'NONE', *, *, #472, .T. ) ;
#9022=ORIENTED_EDGE ( 'NONE', *, *, #3792, .F. ) ;
#9026=DIRECTION ( 'NONE',  ( 0.000000000000000000, 0.000000000000000000, -1.000000000000000000 ) ) ;
#9028=ORIENTED_EDGE ( 'NONE', *, *, #493, .F. ) ;
#9035=DIRECTION ( 'NONE',  ( -0.9578262852211513190, 0.2873478855663453846, 0.000000000000000000 ) ) ;
#9037=DIRECTION ( 'NONE',  ( 1.000000000000000000, 0.000000000000000000, 0.000000000000000000 ) ) ;
#9044=ORIENTED_EDGE ( 'NONE', *, *, #3411, .F. ) ;
#9050=EDGE_CURVE ( 'NONE', #2847, #145, #12187, .T. ) ;
#9062=ORIENTED_EDGE ( 'NONE', *, *, #3792, .T. ) ;
#9064=CARTESIAN_POINT ( 'NONE',  ( 10.00000000000000000, 10.00000000000000178, 210.0000000000000000 ) ) ;
#9068=DIRECTION ( 'NONE',  ( -0.000000000000000000, -0.000000000000000000, 1.000000000000000000 ) ) ;
#9074=DIRECTION ( 'NONE',  ( -1.000000000000000000, 0.000000000000000000, 0.000000000000000000 ) ) ;
#9077=ORIENTED_EDGE ( 'NONE', *, *, #10389, .F. ) ;
#9080=VERTEX_POINT ( 'NONE', #1871 ) ;
#9085=EDGE_CURVE ( 'NONE', #9145, #8805, #1208, .T. ) ;
#9086=FACE_OUTER_BOUND ( 'NONE', #9304, .T. ) ;
#9094=CARTESIAN_POINT ( 'NONE',  ( 451.3035746174796827, 294.6698471414878782, 210.0000000000000000 ) ) ;
#9105=PLANE ( 'NONE',  #12428 ) ;
#9115=EDGE_CURVE ( 'NONE', #5721, #8820, #13100, .T. ) ;
#9120=LINE ( 'NONE', #13489, #3057 ) ;
#9122=CARTESIAN_POINT ( 'NONE',  ( 446.3084422793565409, 264.0194060144110608, 187.0000000000000000 ) ) ;
#9124=VECTOR ( 'NONE', #3180, 1000.000000000000000 ) ;
#9130=CARTESIAN_POINT ( 'NONE',  ( 639.6003227092664929, 153.9938615730590641, -210.0000000000000284 ) ) ;
#9145=VERTEX_POINT ( 'NONE', #3488 ) ;
#9147=VECTOR ( 'NONE', #5410, 1000.000000000000000 ) ;
#9149=ORIENTED_EDGE ( 'NONE', *, *, #2675, .F. ) ;
#9151=DIRECTION ( 'NONE',  ( -0.000000000000000000, -0.000000000000000000, 1.000000000000000000 ) ) ;
#9161=DIRECTION ( 'NONE',  ( -0.000000000000000000, -0.000000000000000000, 1.000000000000000000 ) ) ;
#9168=CARTESIAN_POINT ( 'NONE',  ( 633.0368908673052601, 152.6952049249875927, 210.0000119999999981 ) ) ;
#9170=AXIS2_PLACEMENT_3D ( 'NONE', #14077, #624, #13939 ) ;
#9179=CARTESIAN_POINT ( 'NONE',  ( 145.1678582058265192, 408.6511750828049117, 210.0000000000000000 ) ) ;
#9191=EDGE_CURVE ( 'NONE', #5769, #12523, #10133, .T. ) ;
#9192=CIRCLE ( 'NONE', #1877, 5.249999999999976907 ) ;
#9194=VECTOR ( 'NONE', #4460, 1000.000000000000114 ) ;
#9202=LINE ( 'NONE', #10086, #13133 ) ;
#9205=ORIENTED_EDGE ( 'NONE', *, *, #9433, .F. ) ;
#9215=DIRECTION ( 'NONE',  ( 0.000000000000000000, 0.000000000000000000, -1.000000000000000000 ) ) ;
#9216=VECTOR ( 'NONE', #13209, 1000.000000000000000 ) ;
#9219=LINE ( 'NONE', #4807, #8059 ) ;
#9221=VECTOR ( 'NONE', #11358, 1000.000000000000000 ) ;
#9230=VECTOR ( 'NONE', #6412, 1000.000000000000000 ) ;
#9233=ORIENTED_EDGE ( 'NONE', *, *, #11131, .T. ) ;
#9238=AXIS2_PLACEMENT_3D ( 'NONE', #6093, #10595, #1451 ) ;
#9261=DIRECTION ( 'NONE',  ( 0.000000000000000000, -1.000000000000000000, 0.000000000000000000 ) ) ;
#9272=VECTOR ( 'NONE', #8868, 1000.000000000000000 ) ;
#9276=VERTEX_POINT ( 'NONE', #2454 ) ;
#9296=ORIENTED_EDGE ( 'NONE', *, *, #5824, .F. ) ;
#9301=VERTEX_POINT ( 'NONE', #217 ) ;
#9303=VERTEX_POINT ( 'NONE', #11523 ) ;
#9304=EDGE_LOOP ( 'NONE', ( #7325, #1262, #4816, #11989 ) ) ;
#9313=CARTESIAN_POINT ( 'NONE',  ( 610.0000000000000000, 227.4403065089105951, 190.0000000000000000 ) ) ;
#9321=ORIENTED_EDGE ( 'NONE', *, *, #347, .T. ) ;
#9322=CARTESIAN_POINT ( 'NONE',  ( 638.7771423527817660, 153.4466020873429954, 210.0000119999999981 ) ) ;
#9358=DIRECTION ( 'NONE',  ( 0.000000000000000000, 0.000000000000000000, -1.000000000000000000 ) ) ;
#9363=CARTESIAN_POINT ( 'NONE',  ( 152.8304684875957378, 364.5911659626319192, 210.0000000000000000 ) ) ;
#9387=CARTESIAN_POINT ( 'NONE',  ( 0.000000000000000000, 0.000000000000000000, 210.0000000000000000 ) ) ;
#9392=CARTESIAN_POINT ( 'NONE',  ( 642.5000000000001137, 160.0000000000000284, 210.0000059999999849 ) ) ;
#9403=LINE ( 'NONE', #10362, #13849 ) ;
#9411=CARTESIAN_POINT ( 'NONE',  ( 112.9652219749295341, 376.5507399164317803, -190.0000000000000000 ) ) ;
#9433=EDGE_CURVE ( 'NONE', #1936, #2990, #2517, .T. ) ;
#9434=AXIS2_PLACEMENT_3D ( 'NONE', #12355, #1290, #82 ) ;
#9440=AXIS2_PLACEMENT_3D ( 'NONE', #4347, #14302, #6417 ) ;
#9452=ORIENTED_EDGE ( 'NONE', *, *, #2264, .F. ) ;
#9454=DIRECTION ( 'NONE',  ( 0.000000000000000000, 0.000000000000000000, -1.000000000000000000 ) ) ;
#9455=( GEOMETRIC_REPRESENTATION_CONTEXT ( 3 ) GLOBAL_UNCERTAINTY_ASSIGNED_CONTEXT ( ( #11224 ) ) GLOBAL_UNIT_ASSIGNED_CONTEXT ( ( #851, #5371, #12006 ) ) REPRESENTATION_CONTEXT ( 'NONE', 'WORKASPACE' ) );
#9457=FACE_OUTER_BOUND ( 'NONE', #9500, .T. ) ;
#9459=DIRECTION ( 'NONE',  ( 0.000000000000000000, -1.000000000000000000, 0.000000000000000000 ) ) ;
#9464=VECTOR ( 'NONE', #7805, 1000.000000000000114 ) ;
#9467=CARTESIAN_POINT ( 'NONE',  ( 629.7500000000000000, 160.0000000000000284, -207.0000000000000000 ) ) ;
#9473=VERTEX_POINT ( 'NONE', #1996 ) ;
#9482=VECTOR ( 'NONE', #413, 1000.000000000000114 ) ;
#9487=LINE ( 'NONE', #8211, #10074 ) ;
#9489=ORIENTED_EDGE ( 'NONE', *, *, #1499, .F. ) ;
#9490=AXIS2_PLACEMENT_3D ( 'NONE', #10027, #7470, #8511 ) ;
#9493=ORIENTED_EDGE ( 'NONE', *, *, #3711, .T. ) ;
#9500=EDGE_LOOP ( 'NONE', ( #10492, #5163, #9678, #1062 ) ) ;
#9505=ORIENTED_EDGE ( 'NONE', *, *, #14037, .T. ) ;
#9514=LINE ( 'NONE', #7501, #13424 ) ;
#9534=LINE ( 'NONE', #3921, #11562 ) ;
#9536=ORIENTED_EDGE ( 'NONE', *, *, #4371, .T. ) ;
#9542=VERTEX_POINT ( 'NONE', #4004 ) ;
#9547=EDGE_CURVE ( 'NONE', #5965, #6145, #13677, .T. ) ;
#9548=EDGE_CURVE ( 'NONE', #14559, #4861, #7402, .T. ) ;
#9549=DIRECTION ( 'NONE',  ( -1.000000000000000000, 0.000000000000000000, 0.000000000000000000 ) ) ;
#9556=CARTESIAN_POINT ( 'NONE',  ( 164.3243839102495656, 402.9042173714779551, 210.0000000000000000 ) ) ;
#9563=LINE ( 'NONE', #606, #3096 ) ;
#9564=EDGE_CURVE ( 'NONE', #14011, #7999, #4222, .T. ) ;
#9567=DIRECTION ( 'NONE',  ( -1.000000000000000000, 0.000000000000000000, 0.000000000000000000 ) ) ;
#9568=ORIENTED_EDGE ( 'NONE', *, *, #6073, .F. ) ;
#9569=CARTESIAN_POINT ( 'NONE',  ( 107.2182642636026202, 357.3942142120087055, 210.0000000000000000 ) ) ;
#9577=ORIENTED_EDGE ( 'NONE', *, *, #1124, .F. ) ;
#9581=CARTESIAN_POINT ( 'NONE',  ( 629.7500000000000000, 160.0000000000000284, 207.0000000000000000 ) ) ;
#9586=FACE_OUTER_BOUND ( 'NONE', #8218, .T. ) ;
#9598=LINE ( 'NONE', #11722, #7678 ) ;
#9599=VERTEX_POINT ( 'NONE', #9765 ) ;
#9601=LINE ( 'NONE', #804, #2562 ) ;
#9607=ORIENTED_EDGE ( 'NONE', *, *, #13158, .T. ) ;
#9612=EDGE_CURVE ( 'NONE', #1794, #3289, #8645, .T. ) ;
#9616=VECTOR ( 'NONE', #10143, 1000.000000000000114 ) ;
#9620=EDGE_CURVE ( 'NONE', #10129, #3017, #12246, .T. ) ;
#9621=LINE ( 'NONE', #11676, #14336 ) ;
#9631=VECTOR ( 'NONE', #10094, 1000.000000000000114 ) ;
#9638=FACE_BOUND ( 'NONE', #6515, .T. ) ;
#9639=CARTESIAN_POINT ( 'NONE',  ( 152.8304684875957378, 364.5911659626319192, -210.0000000000000000 ) ) ;
#9641=VECTOR ( 'NONE', #9986, 1000.000000000000000 ) ;
#9649=CARTESIAN_POINT ( 'NONE',  ( 443.6584422793565636, 264.0194060144110608, 210.0000000000000000 ) ) ;
#9651=ORIENTED_EDGE ( 'NONE', *, *, #130, .T. ) ;
#9652=ADVANCED_FACE ( 'NONE', ( #10038 ), #2276, .F. ) ;
#9664=CARTESIAN_POINT ( 'NONE',  ( 627.5000000000000000, 160.0000000000000284, 210.0000119999999981 ) ) ;
#9666=AXIS2_PLACEMENT_3D ( 'NONE', #6046, #7008, #8335 ) ;
#9675=CARTESIAN_POINT ( 'NONE',  ( 10.00000000000000000, 10.00000000000000178, 210.0000000000000000 ) ) ;
#9678=ORIENTED_EDGE ( 'NONE', *, *, #1428, .F. ) ;
#9679=AXIS2_PLACEMENT_3D ( 'NONE', #10993, #3115, #6438 ) ;
#9690=DIRECTION ( 'NONE',  ( -0.000000000000000000, -0.000000000000000000, -1.000000000000000000 ) ) ;
#9691=EDGE_CURVE ( 'NONE', #11174, #8728, #2354, .T. ) ;
#9708=EDGE_LOOP ( 'NONE', ( #7919, #11455, #2098, #10989, #8841, #7160, #10665, #13449, #1205, #13713, #6615, #10290, #11599, #6224, #14394, #8187, #10168, #12540, #750, #3076 ) ) ;
#9720=CARTESIAN_POINT ( 'NONE',  ( 630.3908996001882770, 165.9975013179864618, 210.0000119999999981 ) ) ;
#9725=EDGE_LOOP ( 'NONE', ( #9044, #5575, #14219, #8111 ) ) ;
#9728=ORIENTED_EDGE ( 'NONE', *, *, #5928, .F. ) ;
#9734=ADVANCED_FACE ( 'NONE', ( #1265 ), #10264, .F. ) ;
#9736=ORIENTED_EDGE ( 'NONE', *, *, #4446, .T. ) ;
#9744=EDGE_LOOP ( 'NONE', ( #13222, #14438, #12105, #12 ) ) ;
#9747=DIRECTION ( 'NONE',  ( -0.9578262852211513190, 0.2873478855663453846, 0.000000000000000000 ) ) ;
#9763=EDGE_LOOP ( 'NONE', ( #3371, #10092, #8441, #180 ) ) ;
#9765=CARTESIAN_POINT ( 'NONE',  ( 590.0000000000000000, 212.5596934910894333, 210.0000000000000000 ) ) ;
#9772=EDGE_CURVE ( 'NONE', #5212, #8286, #1182, .T. ) ;
#9783=ORIENTED_EDGE ( 'NONE', *, *, #6189, .T. ) ;
#9790=DIRECTION ( 'NONE',  ( -1.000000000000000000, 0.000000000000000000, 0.000000000000000000 ) ) ;
#9797=VERTEX_POINT ( 'NONE', #11505 ) ;
#9800=DIRECTION ( 'NONE',  ( -0.000000000000000000, -0.000000000000000000, -1.000000000000000000 ) ) ;
#9801=CARTESIAN_POINT ( 'NONE',  ( 153.1991633467111456, 386.6211705227183870, 210.0000000000000000 ) ) ;
#9817=ORIENTED_EDGE ( 'NONE', *, *, #13661, .T. ) ;
#9823=FACE_OUTER_BOUND ( 'NONE', #2723, .T. ) ;
#9845=VECTOR ( 'NONE', #3768, 1000.000000000000000 ) ;
#9855=AXIS2_PLACEMENT_3D ( 'NONE', #10867, #7244, #11731 ) ;
#9860=DIRECTION ( 'NONE',  ( 0.9578262852211514300, -0.2873478855663454401, 0.000000000000000000 ) ) ;
#9876=VERTEX_POINT ( 'NONE', #4226 ) ;
#9881=CARTESIAN_POINT ( 'NONE',  ( 627.6903011687218168, 161.9515302464737943, -210.0000000000000000 ) ) ;
#9883=EDGE_CURVE ( 'NONE', #1138, #5518, #5669, .T. ) ;
#9895=ORIENTED_EDGE ( 'NONE', *, *, #6752, .T. ) ;
#9922=AXIS2_PLACEMENT_3D ( 'NONE', #441, #4971, #213 ) ;
#9926=LINE ( 'NONE', #12058, #4042 ) ;
#9928=AXIS2_PLACEMENT_3D ( 'NONE', #4565, #8900, #3381 ) ;
#9929=EDGE_LOOP ( 'NONE', ( #13977, #4021 ) ) ;
#9930=FACE_BOUND ( 'NONE', #5587, .T. ) ;
#9938=VECTOR ( 'NONE', #10972, 1000.000000000000000 ) ;
#9946=CARTESIAN_POINT ( 'NONE',  ( 610.0000000000000000, 175.0000000000000568, -210.0000000000000000 ) ) ;
#9947=DIRECTION ( 'NONE',  ( 0.000000000000000000, 0.000000000000000000, 1.000000000000000000 ) ) ;
#9949=ORIENTED_EDGE ( 'NONE', *, *, #5113, .T. ) ;
#9950=DIRECTION ( 'NONE',  ( -0.9578262852211513190, 0.2873478855663453846, 0.000000000000000000 ) ) ;
#9959=ORIENTED_EDGE ( 'NONE', *, *, #11307, .T. ) ;
#9961=CARTESIAN_POINT ( 'NONE',  ( 133.6739427831727198, 370.3381236739588758, 210.0000000000000000 ) ) ;
#9964=CARTESIAN_POINT ( 'NONE',  ( 610.0000000000000000, 145.0000000000000568, -190.0000000000000000 ) ) ;
#9968=ORIENTED_EDGE ( 'NONE', *, *, #11668, .T. ) ;
#9969=CARTESIAN_POINT ( 'NONE',  ( 455.5035746174796714, 294.6698471414878782, 210.0000000000000000 ) ) ;
#9974=ORIENTED_EDGE ( 'NONE', *, *, #9115, .T. ) ;
#9979=ORIENTED_EDGE ( 'NONE', *, *, #5569, .F. ) ;
#9986=DIRECTION ( 'NONE',  ( -0.000000000000000000, -0.000000000000000000, 1.000000000000000000 ) ) ;
#10006=EDGE_LOOP ( 'NONE', ( #2658, #6371 ) ) ;
#10012=DIRECTION ( 'NONE',  ( 0.000000000000000000, 0.000000000000000000, 1.000000000000000000 ) ) ;
#10019=ADVANCED_FACE ( 'NONE', ( #9086 ), #12693, .F. ) ;
#10020=ORIENTED_EDGE ( 'NONE', *, *, #791, .T. ) ;
#10027=CARTESIAN_POINT ( 'NONE',  ( 455.5035746174796714, 294.6698471414878782, -210.0000000000000000 ) ) ;
#10033=PRODUCT_CONTEXT ( 'NONE', #14428, 'mechanical' ) ;
#10038=FACE_OUTER_BOUND ( 'NONE', #7583, .T. ) ;
#10042=EDGE_LOOP ( 'NONE', ( #9607, #7727, #12638, #9651 ) ) ;
#10043=LINE ( 'NONE', #2282, #13034 ) ;
#10044=VERTEX_POINT ( 'NONE', #1183 ) ;
#10045=LINE ( 'NONE', #6518, #9147 ) ;
#10046=DIRECTION ( 'NONE',  ( 1.000000000000000000, 0.000000000000000000, 0.000000000000000000 ) ) ;
#10059=AXIS2_PLACEMENT_3D ( 'NONE', #1798, #11906, #12953 ) ;
#10062=CARTESIAN_POINT ( 'NONE',  ( 610.0000000000000000, 145.0000000000000568, 190.0000000000000000 ) ) ;
#10068=EDGE_CURVE ( 'NONE', #12479, #7181, #13586, .T. ) ;
#10069=DIRECTION ( 'NONE',  ( -0.2873478855663453846, -0.9578262852211513190, -0.000000000000000000 ) ) ;
#10070=VERTEX_POINT ( 'NONE', #2444 ) ;
#10074=VECTOR ( 'NONE', #11612, 1000.000000000000000 ) ;
#10078=DIRECTION ( 'NONE',  ( 0.000000000000000000, 0.000000000000000000, -1.000000000000000000 ) ) ;
#10079=ORIENTED_EDGE ( 'NONE', *, *, #11307, .F. ) ;
#10085=VECTOR ( 'NONE', #5718, 1000.000000000000000 ) ;
#10086=CARTESIAN_POINT ( 'NONE',  ( -9.498873539028489220E-16, 10.00000000000000000, -210.0000000000000000 ) ) ;
#10090=EDGE_CURVE ( 'NONE', #54, #14275, #1267, .T. ) ;
#10092=ORIENTED_EDGE ( 'NONE', *, *, #10433, .F. ) ;
#10094=DIRECTION ( 'NONE',  ( -0.9578262852211513190, 0.2873478855663453846, 0.000000000000000000 ) ) ;
#10100=CARTESIAN_POINT ( 'NONE',  ( 451.3035746174797396, 294.6698471414878782, -190.0000000000000000 ) ) ;
#10104=ORIENTED_EDGE ( 'NONE', *, *, #2136, .T. ) ;
#10123=CYLINDRICAL_SURFACE ( 'NONE', #2078, 4.199999999999926459 ) ;
#10127=CIRCLE ( 'NONE', #1416, 7.500000000000062172 ) ;
#10128=EDGE_CURVE ( 'NONE', #1845, #4375, #3990, .T. ) ;
#10129=VERTEX_POINT ( 'NONE', #9675 ) ;
#10133=CIRCLE ( 'NONE', #6410, 5.249999999999976907 ) ;
#10135=FACE_OUTER_BOUND ( 'NONE', #7702, .T. ) ;
#10143=DIRECTION ( 'NONE',  ( -0.2873478855663453846, -0.9578262852211513190, -0.000000000000000000 ) ) ;
#10147=ORIENTED_EDGE ( 'NONE', *, *, #1242, .T. ) ;
#10149=DIRECTION ( 'NONE',  ( 1.000000000000000000, 0.000000000000000000, -0.000000000000000000 ) ) ;
#10151=ORIENTED_EDGE ( 'NONE', *, *, #8270, .F. ) ;
#10157=CARTESIAN_POINT ( 'NONE',  ( 148.9991633467111569, 386.6211705227183870, 190.0000000000000000 ) ) ;
#10158=AXIS2_PLACEMENT_3D ( 'NONE', #4421, #6565, #12161 ) ;
#10164=CARTESIAN_POINT ( 'NONE',  ( 137.1540310085880776, 355.9707293956415697, 210.0000000000000000 ) ) ;
#10167=EDGE_CURVE ( 'NONE', #9876, #11914, #10636, .T. ) ;
#10168=ORIENTED_EDGE ( 'NONE', *, *, #13661, .F. ) ;
#10171=CIRCLE ( 'NONE', #2142, 2.649999999999985700 ) ;
#10183=DIRECTION ( 'NONE',  ( -0.9578262852211513190, 0.2873478855663453846, 0.000000000000000000 ) ) ;
#10187=ORIENTED_EDGE ( 'NONE', *, *, #5569, .T. ) ;
#10193=ORIENTED_EDGE ( 'NONE', *, *, #4905, .F. ) ;
#10194=VERTEX_POINT ( 'NONE', #6050 ) ;
#10195=AXIS2_PLACEMENT_3D ( 'NONE', #499, #12902, #12758 ) ;
#10201=VECTOR ( 'NONE', #6552, 1000.000000000000000 ) ;
#10206=LINE ( 'NONE', #7978, #1378 ) ;
#10207=EDGE_CURVE ( 'NONE', #4375, #14524, #9534, .T. ) ;
#10210=VERTEX_POINT ( 'NONE', #10554 ) ;
#10216=EDGE_CURVE ( 'NONE', #5721, #6493, #7305, .T. ) ;
#10221=DIRECTION ( 'NONE',  ( -0.000000000000000000, -0.000000000000000000, -1.000000000000000000 ) ) ;
#10224=LINE ( 'NONE', #5570, #13665 ) ;
#10227=CARTESIAN_POINT ( 'NONE',  ( -10.00000000000000000, 413.4403065089105667, -190.0000000000000000 ) ) ;
#10228=VERTEX_POINT ( 'NONE', #8405 ) ;
#10229=DIRECTION ( 'NONE',  ( 1.000000000000000000, 0.000000000000000000, 0.000000000000000000 ) ) ;
#10231=CARTESIAN_POINT ( 'NONE',  ( 455.5035746174796714, 294.6698471414878782, 210.0000000000000000 ) ) ;
#10232=ORIENTED_EDGE ( 'NONE', *, *, #9620, .T. ) ;
#10236=( NAMED_UNIT ( * ) SI_UNIT ( $, .STERADIAN. ) SOLID_ANGLE_UNIT ( ) );
#10239=ORIENTED_EDGE ( 'NONE', *, *, #2130, .F. ) ;
#10246=CARTESIAN_POINT ( 'NONE',  ( 627.5000000000000000, 160.0000000000000284, -210.0000059999999849 ) ) ;
#10249=CARTESIAN_POINT ( 'NONE',  ( 590.0000000000000000, 10.00000000000005507, 190.0000000000000000 ) ) ;
#10258=EDGE_LOOP ( 'NONE', ( #12199, #5311 ) ) ;
#10260=EDGE_CURVE ( 'NONE', #2949, #10957, #4265, .T. ) ;
#10264=CYLINDRICAL_SURFACE ( 'NONE', #5434, 4.199999999999926459 ) ;
#10267=CARTESIAN_POINT ( 'NONE',  ( 610.0000000000000000, 0.000000000000000000, -190.0000000000000000 ) ) ;
#10272=LINE ( 'NONE', #132, #11272 ) ;
#10278=CARTESIAN_POINT ( 'NONE',  ( 636.9631091326946262, 152.6952049249875927, 210.0000119999999981 ) ) ;
#10280=CARTESIAN_POINT ( 'NONE',  ( 610.0000000000000000, 10.00000000000005507, 190.0000000000000000 ) ) ;
#10281=FACE_BOUND ( 'NONE', #13793, .T. ) ;
#10288=FACE_OUTER_BOUND ( 'NONE', #7622, .T. ) ;
#10290=ORIENTED_EDGE ( 'NONE', *, *, #8876, .F. ) ;
#10296=DIRECTION ( 'NONE',  ( 1.000000000000000000, 0.000000000000000000, 0.000000000000000000 ) ) ;
#10298=LINE ( 'NONE', #165, #3832 ) ;
#10299=CARTESIAN_POINT ( 'NONE',  ( 629.7500000000000000, 160.0000000000000284, 190.0000000000000284 ) ) ;
#10309=ADVANCED_FACE ( 'NONE', ( #7524 ), #12229, .F. ) ;
#10313=FACE_OUTER_BOUND ( 'NONE', #9744, .T. ) ;
#10316=LINE ( 'NONE', #265, #9221 ) ;
#10341=FACE_BOUND ( 'NONE', #12618, .T. ) ;
#10348=CARTESIAN_POINT ( 'NONE',  ( 634.0182522957532001, 152.5000000000000000, 210.0000120000000265 ) ) ;
#10350=CIRCLE ( 'NONE', #12219, 2.649999999999985700 ) ;
#10356=VERTEX_POINT ( 'NONE', #9964 ) ;
#10360=AXIS2_PLACEMENT_3D ( 'NONE', #1145, #26, #6835 ) ;
#10362=CARTESIAN_POINT ( 'NONE',  ( 9.498873539028489220E-16, -10.00000000000000000, -210.0000000000000000 ) ) ;
#10371=VECTOR ( 'NONE', #7928, 1000.000000000000000 ) ;
#10378=DIRECTION ( 'NONE',  ( 0.2873478855663453846, 0.9578262852211513190, 0.000000000000000000 ) ) ;
#10379=CIRCLE ( 'NONE', #8253, 2.649999999999985700 ) ;
#10386=AXIS2_PLACEMENT_3D ( 'NONE', #3540, #5891, #6775 ) ;
#10389=EDGE_CURVE ( 'NONE', #11414, #12665, #2047, .T. ) ;
#10393=AXIS2_PLACEMENT_3D ( 'NONE', #1064, #9860, #8609 ) ;
#10394=CARTESIAN_POINT ( 'NONE',  ( 641.0062790085321467, 155.3995367091426658, -210.0000000000000000 ) ) ;
#10395=CARTESIAN_POINT ( 'NONE',  ( 152.8304684875957378, 364.5911659626319192, -210.0000000000000000 ) ) ;
#10409=VECTOR ( 'NONE', #922, 1000.000000000000114 ) ;
#10410=DIRECTION ( 'NONE',  ( -1.000000000000000000, 0.000000000000000000, 0.000000000000000000 ) ) ;
#10417=AXIS2_PLACEMENT_3D ( 'NONE', #9569, #10676, #550 ) ;
#10418=EDGE_CURVE ( 'NONE', #5518, #1138, #6871, .T. ) ;
#10431=CARTESIAN_POINT ( 'NONE',  ( 139.8040310085880833, 355.9707293956415697, -190.0000000000000000 ) ) ;
#10433=EDGE_CURVE ( 'NONE', #6145, #5965, #10171, .T. ) ;
#10448=VERTEX_POINT ( 'NONE', #5596 ) ;
#10452=CLOSED_SHELL ( 'NONE', ( #12159, #871, #11952, #3938, #12289, #9734, #2404, #2868, #5574, #594, #11689, #3898, #12750, #5017, #2460, #5676, #1484, #3479, #8148, #8150, #5155, #11990, #4601, #10019, #7369, #6694, #13583, #4998, #3330, #14064, #12426, #11037, #7313, #6947, #10707, #3041, #11175, #4664, #7643, #4033, #7510, #5387, #5793, #6942, #8682, #1872, #8598, #13079, #1066, #10495, #2344, #14410, #9652, #13772, #819, #8031, #2503, #10889, #6561, #3659, #7987, #11780, #13214, #4806, #2341, #14310, #10309, #12594, #7597, #8896, #4866, #13371, #6478 ) ) ;
#10461=EDGE_CURVE ( 'NONE', #4023, #10210, #4504, .T. ) ;
#10470=VERTEX_POINT ( 'NONE', #10246 ) ;
#10482=DIRECTION ( 'NONE',  ( 0.000000000000000000, 0.000000000000000000, 1.000000000000000000 ) ) ;
#10486=ORIENTED_EDGE ( 'NONE', *, *, #4324, .F. ) ;
#10488=FACE_BOUND ( 'NONE', #13190, .T. ) ;
#10492=ORIENTED_EDGE ( 'NONE', *, *, #4714, .T. ) ;
#10495=ADVANCED_FACE ( 'NONE', ( #13638 ), #5677, .F. ) ;
#10499=DIRECTION ( 'NONE',  ( -0.000000000000000000, -0.000000000000000000, 1.000000000000000000 ) ) ;
#10502=CARTESIAN_POINT ( 'NONE',  ( 590.0000000000000000, 212.5596934910894333, 190.0000000000000000 ) ) ;
#10509=VERTEX_POINT ( 'NONE', #10100 ) ;
#10512=EDGE_CURVE ( 'NONE', #7886, #1138, #105, .T. ) ;
#10513=LINE ( 'NONE', #14065, #8496 ) ;
#10515=DIRECTION ( 'NONE',  ( 0.9578262852211515410, -0.2873478855663446074, 0.000000000000000000 ) ) ;
#10517=VERTEX_POINT ( 'NONE', #2487 ) ;
#10529=DIRECTION ( 'NONE',  ( 0.000000000000000000, -1.000000000000000000, -0.000000000000000000 ) ) ;
#10530=EDGE_CURVE ( 'NONE', #4698, #10517, #10316, .T. ) ;
#10532=CARTESIAN_POINT ( 'NONE',  ( 112.9652219749295341, 376.5507399164317803, 190.0000000000000000 ) ) ;
#10540=ORIENTED_EDGE ( 'NONE', *, *, #7922, .T. ) ;
#10554=CARTESIAN_POINT ( 'NONE',  ( -10.00000000000000000, 413.4403065089105667, 210.0000000000000000 ) ) ;
#10557=AXIS2_PLACEMENT_3D ( 'NONE', #10649, #13083, #4003 ) ;
#10562=DIRECTION ( 'NONE',  ( -0.9578262852211513190, 0.2873478855663453846, 0.000000000000000000 ) ) ;
#10565=DIRECTION ( 'NONE',  ( -0.000000000000000000, -0.000000000000000000, -1.000000000000000000 ) ) ;
#10571=DIRECTION ( 'NONE',  ( -0.000000000000000000, -0.000000000000000000, -1.000000000000000000 ) ) ;
#10578=LINE ( 'NONE', #2749, #6563 ) ;
#10579=DIRECTION ( 'NONE',  ( 0.000000000000000000, 0.000000000000000000, 1.000000000000000000 ) ) ;
#10585=VERTEX_POINT ( 'NONE', #12899 ) ;
#10589=DIRECTION ( 'NONE',  ( -0.2873478855663453846, -0.9578262852211513190, -0.000000000000000000 ) ) ;
#10591=VECTOR ( 'NONE', #12691, 1000.000000000000000 ) ;
#10595=DIRECTION ( 'NONE',  ( 0.000000000000000000, 0.000000000000000000, 1.000000000000000000 ) ) ;
#10599=CARTESIAN_POINT ( 'NONE',  ( 112.9652219749295341, 376.5507399164317803, -210.0000000000000000 ) ) ;
#10603=FACE_BOUND ( 'NONE', #1194, .T. ) ;
#10605=ORIENTED_EDGE ( 'NONE', *, *, #13985, .T. ) ;
#10608=EDGE_CURVE ( 'NONE', #7099, #14275, #10615, .T. ) ;
#10615=LINE ( 'NONE', #12976, #10648 ) ;
#10625=VECTOR ( 'NONE', #3780, 1000.000000000000000 ) ;
#10633=EDGE_CURVE ( 'NONE', #9276, #9473, #6032, .T. ) ;
#10636=LINE ( 'NONE', #12997, #2378 ) ;
#10648=VECTOR ( 'NONE', #1752, 1000.000000000000000 ) ;
#10649=CARTESIAN_POINT ( 'NONE',  ( 148.9991633467111569, 386.6211705227183870, -210.0000000000000000 ) ) ;
#10656=VECTOR ( 'NONE', #12865, 1000.000000000000000 ) ;
#10660=EDGE_CURVE ( 'NONE', #197, #542, #3085, .T. ) ;
#10665=ORIENTED_EDGE ( 'NONE', *, *, #10633, .F. ) ;
#10667=DIRECTION ( 'NONE',  ( -1.000000000000000000, 0.000000000000000000, 0.000000000000000000 ) ) ;
#10672=LINE ( 'NONE', #8595, #6840 ) ;
#10674=DIRECTION ( 'NONE',  ( 0.9578262852211514300, -0.2873478855663454401, 0.000000000000000000 ) ) ;
#10675=ORIENTED_EDGE ( 'NONE', *, *, #5211, .T. ) ;
#10676=DIRECTION ( 'NONE',  ( -0.2873478855663454401, -0.9578262852211514300, 0.000000000000000000 ) ) ;
#10682=CARTESIAN_POINT ( 'NONE',  ( 610.0000000000000000, 10.00000000000005507, 190.0000000000000000 ) ) ;
#10707=ADVANCED_FACE ( 'NONE', ( #7728 ), #10832, .F. ) ;
#10724=EDGE_CURVE ( 'NONE', #1544, #11118, #5696, .T. ) ;
#10737=CARTESIAN_POINT ( 'NONE',  ( 635.0000000000000000, 160.0000000000000284, -207.0000000000000000 ) ) ;
#10742=CARTESIAN_POINT ( 'NONE',  ( 640.9975013179864618, 164.6091003998119788, 210.0000120000000265 ) ) ;
#10746=FACE_BOUND ( 'NONE', #74, .T. ) ;
#10766=CARTESIAN_POINT ( 'NONE',  ( 641.5487773412237402, 163.7885571598201579, -209.9999999999999432 ) ) ;
#10771=DIRECTION ( 'NONE',  ( 0.000000000000000000, 0.000000000000000000, -1.000000000000000000 ) ) ;
#10779=CIRCLE ( 'NONE', #10059, 5.249999999999976907 ) ;
#10794=CARTESIAN_POINT ( 'NONE',  ( 590.0000000000000000, 10.00000000000005507, -190.0000000000000000 ) ) ;
#10798=DIRECTION ( 'NONE',  ( 0.000000000000000000, 0.000000000000000000, 1.000000000000000000 ) ) ;
#10804=AXIS2_PLACEMENT_3D ( 'NONE', #1985, #7819, #2197 ) ;
#10814=CARTESIAN_POINT ( 'NONE',  ( 10.00000000000000000, -10.00000000000000000, -190.0000000000000000 ) ) ;
#10815=CARTESIAN_POINT ( 'NONE',  ( 635.9817477042469136, 167.5000000000000853, 210.0000120000000265 ) ) ;
#10821=ORIENTED_EDGE ( 'NONE', *, *, #9691, .F. ) ;
#10830=LINE ( 'NONE', #2938, #11809 ) ;
#10831=VERTEX_POINT ( 'NONE', #2410 ) ;
#10832=PLANE ( 'NONE',  #13241 ) ;
#10835=EDGE_CURVE ( 'NONE', #8286, #5212, #1679, .T. ) ;
#10836=FACE_OUTER_BOUND ( 'NONE', #12505, .T. ) ;
#10839=VECTOR ( 'NONE', #13721, 1000.000000000000000 ) ;
#10851=AXIS2_PLACEMENT_3D ( 'NONE', #12511, #11406, #1294 ) ;
#10867=CARTESIAN_POINT ( 'NONE',  ( 650.0000000000000000, 145.0000000000000568, -210.0000000000000000 ) ) ;
#10879=DIRECTION ( 'NONE',  ( -0.000000000000000000, -0.000000000000000000, -1.000000000000000000 ) ) ;
#10886=ORIENTED_EDGE ( 'NONE', *, *, #9564, .T. ) ;
#10889=ADVANCED_FACE ( 'NONE', ( #11261 ), #1299, .T. ) ;
#10896=EDGE_CURVE ( 'NONE', #6340, #14092, #14590, .T. ) ;
#10900=EDGE_LOOP ( 'NONE', ( #12293, #7813, #5214, #3618 ) ) ;
#10901=EDGE_CURVE ( 'NONE', #7181, #14510, #10298, .T. ) ;
#10903=DIRECTION ( 'NONE',  ( 0.000000000000000000, 0.000000000000000000, -1.000000000000000000 ) ) ;
#10910=CARTESIAN_POINT ( 'NONE',  ( 144.7991633467111399, 386.6211705227183870, -210.0000000000000000 ) ) ;
#10912=ORIENTED_EDGE ( 'NONE', *, *, #1917, .T. ) ;
#10915=EDGE_CURVE ( 'NONE', #13614, #12303, #976, .T. ) ;
#10917=VECTOR ( 'NONE', #10499, 1000.000000000000000 ) ;
#10923=ORIENTED_EDGE ( 'NONE', *, *, #8891, .T. ) ;
#10925=FACE_OUTER_BOUND ( 'NONE', #12420, .T. ) ;
#10927=CARTESIAN_POINT ( 'NONE',  ( 635.0000000000000000, 160.0000000000000284, -207.0000000000000000 ) ) ;
#10934=LINE ( 'NONE', #8639, #947 ) ;
#10936=ORIENTED_EDGE ( 'NONE', *, *, #12605, .T. ) ;
#10941=ORIENTED_EDGE ( 'NONE', *, *, #10207, .F. ) ;
#10949=ORIENTED_EDGE ( 'NONE', *, *, #12706, .T. ) ;
#10954=EDGE_CURVE ( 'NONE', #3170, #8139, #5243, .T. ) ;
#10957=VERTEX_POINT ( 'NONE', #14069 ) ;
#10972=DIRECTION ( 'NONE',  ( -0.000000000000000000, -0.000000000000000000, -1.000000000000000000 ) ) ;
#10988=CARTESIAN_POINT ( 'NONE',  ( 459.3348797583642522, 272.6398425814014104, 190.0000000000000000 ) ) ;
#10989=ORIENTED_EDGE ( 'NONE', *, *, #13825, .T. ) ;
#10990=CARTESIAN_POINT ( 'NONE',  ( 650.0000000000000000, 175.0000000000000568, -190.0000000000000000 ) ) ;
#10993=CARTESIAN_POINT ( 'NONE',  ( 148.9991633467111569, 386.6211705227183870, -210.0000000000000000 ) ) ;
#11023=VERTEX_POINT ( 'NONE', #2768 ) ;
#11033=ORIENTED_EDGE ( 'NONE', *, *, #10530, .F. ) ;
#11037=ADVANCED_FACE ( 'NONE', ( #7133 ), #6177, .T. ) ;
#11038=CARTESIAN_POINT ( 'NONE',  ( 470.8287951810180516, 310.9528939902474463, 190.0000000000000000 ) ) ;
#11052=ORIENTED_EDGE ( 'NONE', *, *, #10724, .F. ) ;
#11053=CARTESIAN_POINT ( 'NONE',  ( 10.00000000000000000, 386.5596934910894902, -210.0000000000000000 ) ) ;
#11054=LINE ( 'NONE', #937, #8937 ) ;
#11056=VECTOR ( 'NONE', #12070, 1000.000000000000114 ) ;
#11057=CARTESIAN_POINT ( 'NONE',  ( 631.2114428402037447, 166.5487773412478987, -210.0000000000000000 ) ) ;
#11059=CIRCLE ( 'NONE', #9666, 4.199999999999926459 ) ;
#11060=AXIS2_PLACEMENT_3D ( 'NONE', #6068, #10571, #9549 ) ;
#11063=EDGE_CURVE ( 'NONE', #14014, #9797, #1520, .T. ) ;
#11066=DIRECTION ( 'NONE',  ( -1.000000000000000000, -0.000000000000000000, -0.000000000000000000 ) ) ;
#11070=EDGE_CURVE ( 'NONE', #3137, #7506, #8147, .T. ) ;
#11075=CIRCLE ( 'NONE', #6361, 4.200000000000009059 ) ;
#11076=VECTOR ( 'NONE', #2747, 1000.000000000000000 ) ;
#11078=VECTOR ( 'NONE', #1559, 1000.000000000000000 ) ;
#11106=VECTOR ( 'NONE', #3077, 1000.000000000000000 ) ;
#11112=AXIS2_PLACEMENT_3D ( 'NONE', #5517, #10012, #12080 ) ;
#11117=LINE ( 'NONE', #996, #11106 ) ;
#11118=VERTEX_POINT ( 'NONE', #13104 ) ;
#11122=FACE_OUTER_BOUND ( 'NONE', #11481, .T. ) ;
#11124=ORIENTED_EDGE ( 'NONE', *, *, #1124, .T. ) ;
#11131=EDGE_CURVE ( 'NONE', #7099, #11414, #12062, .T. ) ;
#11135=DIRECTION ( 'NONE',  ( -0.000000000000000000, -0.000000000000000000, 1.000000000000000000 ) ) ;
#11137=VECTOR ( 'NONE', #5699, 1000.000000000000000 ) ;
#11141=FACE_OUTER_BOUND ( 'NONE', #5285, .T. ) ;
#11143=CARTESIAN_POINT ( 'NONE',  ( 124.4591373975829214, 414.8637913252775320, 8.883675154640809176E-13 ) ) ;
#11157=ORIENTED_EDGE ( 'NONE', *, *, #8542, .T. ) ;
#11158=EDGE_CURVE ( 'NONE', #8805, #9145, #6172, .T. ) ;
#11162=CARTESIAN_POINT ( 'NONE',  ( 133.6739427831727767, 370.3381236739588189, -190.0000000000000000 ) ) ;
#11173=FACE_OUTER_BOUND ( 'NONE', #14328, .T. ) ;
#11174=VERTEX_POINT ( 'NONE', #14356 ) ;
#11175=ADVANCED_FACE ( 'NONE', ( #4249, #5429, #9930, #9638, #14439, #2167, #11393 ), #4545, .T. ) ;
#11183=CARTESIAN_POINT ( 'NONE',  ( 610.0000000000000000, 175.0000000000000568, -210.0000000000000000 ) ) ;
#11187=ORIENTED_EDGE ( 'NONE', *, *, #5745, .T. ) ;
#11197=ORIENTED_EDGE ( 'NONE', *, *, #5984, .F. ) ;
#11199=ORIENTED_EDGE ( 'NONE', *, *, #3411, .T. ) ;
#11203=CARTESIAN_POINT ( 'NONE',  ( 636.9517704078292581, 167.3095993251051539, -210.0000000000000000 ) ) ;
#11206=CARTESIAN_POINT ( 'NONE',  ( 640.2500000000000000, 160.0000000000000284, -210.0000000000000000 ) ) ;
#11210=DIRECTION ( 'NONE',  ( -0.000000000000000000, -0.000000000000000000, -1.000000000000000000 ) ) ;
#11220=LINE ( 'NONE', #5613, #5637 ) ;
#11224=UNCERTAINTY_MEASURE_WITH_UNIT (LENGTH_MEASURE( 1.000000000000000082E-05 ), #851, 'distance_accuracy_value', 'NONE');
#11226=ORIENTED_EDGE ( 'NONE', *, *, #3407, .T. ) ;
#11227=LINE ( 'NONE', #6878, #3473 ) ;
#11232=ORIENTED_EDGE ( 'NONE', *, *, #14251, .F. ) ;
#11239=CIRCLE ( 'NONE', #4894, 7.500000000000062172 ) ;
#11242=LINE ( 'NONE', #5636, #11076 ) ;
#11248=EDGE_CURVE ( 'NONE', #6071, #5821, #1461, .T. ) ;
#11256=AXIS2_PLACEMENT_3D ( 'NONE', #12134, #3211, #2018 ) ;
#11261=FACE_OUTER_BOUND ( 'NONE', #5010, .T. ) ;
#11264=VECTOR ( 'NONE', #3499, 1000.000000000000000 ) ;
#11272=VECTOR ( 'NONE', #1189, 1000.000000000000000 ) ;
#11284=VECTOR ( 'NONE', #5686, 1000.000000000000114 ) ;
#11303=VECTOR ( 'NONE', #2563, 1000.000000000000114 ) ;
#11307=EDGE_CURVE ( 'NONE', #9876, #14241, #3878, .T. ) ;
#11316=ORIENTED_EDGE ( 'NONE', *, *, #4319, .F. ) ;
#11319=DIRECTION ( 'NONE',  ( 0.000000000000000000, 0.000000000000000000, 1.000000000000000000 ) ) ;
#11331=CIRCLE ( 'NONE', #8506, 4.199999999999926459 ) ;
#11336=LINE ( 'NONE', #11549, #13603 ) ;
#11337=EDGE_CURVE ( 'NONE', #7099, #4375, #11456, .T. ) ;
#11341=AXIS2_PLACEMENT_3D ( 'NONE', #10231, #5729, #10296 ) ;
#11351=LINE ( 'NONE', #9064, #8445 ) ;
#11355=CARTESIAN_POINT ( 'NONE',  ( 448.9584422793565750, 264.0194060144110608, 190.0000000000000000 ) ) ;
#11358=DIRECTION ( 'NONE',  ( -0.000000000000000000, -0.000000000000000000, -1.000000000000000000 ) ) ;
#11363=VERTEX_POINT ( 'NONE', #2973 ) ;
#11373=DIRECTION ( 'NONE',  ( 0.000000000000000000, 0.000000000000000000, -1.000000000000000000 ) ) ;
#11393=FACE_BOUND ( 'NONE', #12218, .T. ) ;
#11406=DIRECTION ( 'NONE',  ( -9.498873539028489960E-17, 1.000000000000000000, 0.000000000000000000 ) ) ;
#11414=VERTEX_POINT ( 'NONE', #7469 ) ;
#11416=ORIENTED_EDGE ( 'NONE', *, *, #4005, .T. ) ;
#11420=CARTESIAN_POINT ( 'NONE',  ( 636.9516943256485320, 152.6905843535471092, -210.0000000000000284 ) ) ;
#11429=DIRECTION ( 'NONE',  ( -0.2873478855663453846, -0.9578262852211513190, 0.000000000000000000 ) ) ;
#11441=DIRECTION ( 'NONE',  ( -0.2873478855663454401, -0.9578262852211514300, 0.000000000000000000 ) ) ;
#11455=ORIENTED_EDGE ( 'NONE', *, *, #2264, .T. ) ;
#11456=LINE ( 'NONE', #12640, #263 ) ;
#11458=EDGE_CURVE ( 'NONE', #3336, #14510, #9219, .T. ) ;
#11477=AXIS2_PLACEMENT_3D ( 'NONE', #9969, #4363, #735 ) ;
#11481=EDGE_LOOP ( 'NONE', ( #6906, #10912, #12876, #12836 ) ) ;
#11484=CARTESIAN_POINT ( 'NONE',  ( 641.5485936625826753, 156.2115189222640197, -210.0000000000000284 ) ) ;
#11487=AXIS2_PLACEMENT_3D ( 'NONE', #2531, #10579, #8293 ) ;
#11488=EDGE_LOOP ( 'NONE', ( #12442, #5263 ) ) ;
#11493=LINE ( 'NONE', #336, #5992 ) ;
#11494=VERTEX_POINT ( 'NONE', #13728 ) ;
#11502=ORIENTED_EDGE ( 'NONE', *, *, #10090, .T. ) ;
#11505=CARTESIAN_POINT ( 'NONE',  ( 10.00000000000000000, 386.5596934910894902, 190.0000000000000000 ) ) ;
#11517=FACE_OUTER_BOUND ( 'NONE', #11645, .T. ) ;
#11523=CARTESIAN_POINT ( 'NONE',  ( 610.0000000000000000, 145.0000000000000568, 210.0000000000000000 ) ) ;
#11526=LINE ( 'NONE', #13676, #2561 ) ;
#11538=ORIENTED_EDGE ( 'NONE', *, *, #3680, .F. ) ;
#11541=ORIENTED_EDGE ( 'NONE', *, *, #5317, .F. ) ;
#11549=CARTESIAN_POINT ( 'NONE',  ( 451.6722694765949768, 316.6998517015743460, 210.0000000000000000 ) ) ;
#11557=ORIENTED_EDGE ( 'NONE', *, *, #8099, .F. ) ;
#11562=VECTOR ( 'NONE', #4963, 1000.000000000000000 ) ;
#11568=MECHANICAL_DESIGN_GEOMETRIC_PRESENTATION_REPRESENTATION('',(#6842),#9455);
#11577=DIRECTION ( 'NONE',  ( 0.9578262852211514300, -0.2873478855663454401, -2.126801590887410810E-15 ) ) ;
#11589=DIRECTION ( 'NONE',  ( -0.2873478855663453846, -0.9578262852211513190, -0.000000000000000000 ) ) ;
#11599=ORIENTED_EDGE ( 'NONE', *, *, #397, .F. ) ;
#11612=DIRECTION ( 'NONE',  ( 0.000000000000000000, 0.000000000000000000, -1.000000000000000000 ) ) ;
#11616=ORIENTED_EDGE ( 'NONE', *, *, #6726, .F. ) ;
#11625=DIRECTION ( 'NONE',  ( 1.000000000000000000, -0.000000000000000000, 0.000000000000000000 ) ) ;
#11630=DIRECTION ( 'NONE',  ( -1.000000000000000000, 0.000000000000000000, 0.000000000000000000 ) ) ;
#11632=ORIENTED_EDGE ( 'NONE', *, *, #9547, .T. ) ;
#11633=PLANE ( 'NONE',  #4713 ) ;
#11635=DIRECTION ( 'NONE',  ( 0.000000000000000000, 0.000000000000000000, -1.000000000000000000 ) ) ;
#11637=PLANE ( 'NONE',  #5449 ) ;
#11638=EDGE_LOOP ( 'NONE', ( #10486, #2824, #1289, #5870 ) ) ;
#11642=DIRECTION ( 'NONE',  ( -1.000000000000000000, 0.000000000000000000, 0.000000000000000000 ) ) ;
#11643=ORIENTED_EDGE ( 'NONE', *, *, #7956, .F. ) ;
#11645=EDGE_LOOP ( 'NONE', ( #9321, #6390, #5050, #393, #9959, #2419, #9895, #1342, #1665, #5894, #4107, #9028, #8739, #7700, #12244, #9949 ) ) ;
#11659=CARTESIAN_POINT ( 'NONE',  ( -10.00000000000000000, 10.00000000000000178, -210.0020000000000095 ) ) ;
#11660=FACE_BOUND ( 'NONE', #14550, .T. ) ;
#11663=ORIENTED_EDGE ( 'NONE', *, *, #14063, .F. ) ;
#11665=LINE ( 'NONE', #2679, #144 ) ;
#11667=DIRECTION ( 'NONE',  ( -0.000000000000000000, -0.000000000000000000, 1.000000000000000000 ) ) ;
#11668=EDGE_CURVE ( 'NONE', #4861, #542, #5088, .T. ) ;
#11676=CARTESIAN_POINT ( 'NONE',  ( 640.2500000000000000, 160.0000000000000284, -210.0000000000000000 ) ) ;
#11681=ORIENTED_EDGE ( 'NONE', *, *, #970, .T. ) ;
#11689=ADVANCED_FACE ( 'NONE', ( #7218 ), #3761, .F. ) ;
#11697=FACE_BOUND ( 'NONE', #10006, .T. ) ;
#11715=ORIENTED_EDGE ( 'NONE', *, *, #13577, .T. ) ;
#11717=VECTOR ( 'NONE', #11758, 1000.000000000000000 ) ;
#11722=CARTESIAN_POINT ( 'NONE',  ( 164.3243839102495656, 402.9042173714779551, 210.0000000000000000 ) ) ;
#11723=VERTEX_POINT ( 'NONE', #9801 ) ;
#11731=DIRECTION ( 'NONE',  ( 0.000000000000000000, -0.000000000000000000, 1.000000000000000000 ) ) ;
#11744=CARTESIAN_POINT ( 'NONE',  ( 112.9652219749295341, 376.5507399164317803, 210.0000000000000000 ) ) ;
#11753=ORIENTED_EDGE ( 'NONE', *, *, #4776, .F. ) ;
#11758=DIRECTION ( 'NONE',  ( 0.000000000000000000, 1.000000000000000000, 0.000000000000000000 ) ) ;
#11760=ORIENTED_EDGE ( 'NONE', *, *, #8876, .T. ) ;
#11765=ORIENTED_EDGE ( 'NONE', *, *, #3686, .F. ) ;
#11770=ORIENTED_EDGE ( 'NONE', *, *, #8165, .T. ) ;
#11774=LINE ( 'NONE', #12825, #6338 ) ;
#11780=ADVANCED_FACE ( 'NONE', ( #10836, #12005 ), #13274, .T. ) ;
#11782=DIRECTION ( 'NONE',  ( -0.9578262852211513190, 0.2873478855663453846, 0.000000000000000000 ) ) ;
#11787=FACE_OUTER_BOUND ( 'NONE', #9725, .T. ) ;
#11794=VECTOR ( 'NONE', #10562, 1000.000000000000114 ) ;
#11795=EDGE_LOOP ( 'NONE', ( #9736, #1732, #3929, #14091 ) ) ;
#11802=FACE_OUTER_BOUND ( 'NONE', #6546, .T. ) ;
#11803=EDGE_CURVE ( 'NONE', #10470, #9145, #4128, .T. ) ;
#11809=VECTOR ( 'NONE', #6190, 1000.000000000000000 ) ;
#11818=AXIS2_PLACEMENT_3D ( 'NONE', #12193, #6242, #14285 ) ;
#11819=DIRECTION ( 'NONE',  ( -0.000000000000000000, -0.000000000000000000, 1.000000000000000000 ) ) ;
#11852=DIRECTION ( 'NONE',  ( 0.000000000000000000, 0.000000000000000000, 1.000000000000000000 ) ) ;
#11856=DIRECTION ( 'NONE',  ( 1.000000000000000000, 0.000000000000000000, 0.000000000000000000 ) ) ;
#11899=EDGE_LOOP ( 'NONE', ( #2376, #13706, #4592, #1438 ) ) ;
#11901=ORIENTED_EDGE ( 'NONE', *, *, #6236, .T. ) ;
#11906=DIRECTION ( 'NONE',  ( -0.000000000000000000, -0.000000000000000000, 1.000000000000000000 ) ) ;
#11908=CARTESIAN_POINT ( 'NONE',  ( 470.8287951810180516, 310.9528939902474463, -190.0000000000000000 ) ) ;
#11911=CARTESIAN_POINT ( 'NONE',  ( 642.5000000000001137, 160.9817477042468568, 210.0000119999999981 ) ) ;
#11913=DIRECTION ( 'NONE',  ( -0.000000000000000000, -0.000000000000000000, -1.000000000000000000 ) ) ;
#11914=VERTEX_POINT ( 'NONE', #13491 ) ;
#11935=VECTOR ( 'NONE', #4710, 1000.000000000000000 ) ;
#11938=MANIFOLD_SOLID_BREP ( 'Mirror13', #10452 ) ;
#11947=CARTESIAN_POINT ( 'NONE',  ( 112.9652219749295341, 376.5507399164317803, 210.0000000000000000 ) ) ;
#11952=ADVANCED_FACE ( 'NONE', ( #12438 ), #4633, .F. ) ;
#11965=ORIENTED_EDGE ( 'NONE', *, *, #11668, .F. ) ;
#11985=CIRCLE ( 'NONE', #9170, 2.649999999999985700 ) ;
#11987=CARTESIAN_POINT ( 'NONE',  ( 470.8287951810180516, 310.9528939902474463, 190.0000000000000000 ) ) ;
#11989=ORIENTED_EDGE ( 'NONE', *, *, #8930, .F. ) ;
#11990=ADVANCED_FACE ( 'NONE', ( #12819 ), #2551, .F. ) ;
#11993=VERTEX_POINT ( 'NONE', #320 ) ;
#11999=CARTESIAN_POINT ( 'NONE',  ( 148.9991633467111569, 386.6211705227183870, 210.0000000000000000 ) ) ;
#12005=FACE_BOUND ( 'NONE', #14140, .T. ) ;
#12006=( NAMED_UNIT ( * ) SI_UNIT ( $, .STERADIAN. ) SOLID_ANGLE_UNIT ( ) );
#12007=ORIENTED_EDGE ( 'NONE', *, *, #3637, .T. ) ;
#12011=ORIENTED_EDGE ( 'NONE', *, *, #6113, .T. ) ;
#12015=DIRECTION ( 'NONE',  ( 1.000000000000000000, 0.000000000000000000, 0.000000000000000000 ) ) ;
#12023=ORIENTED_EDGE ( 'NONE', *, *, #5317, .T. ) ;
#12024=VECTOR ( 'NONE', #1993, 1000.000000000000114 ) ;
#12026=DIRECTION ( 'NONE',  ( -0.000000000000000000, -0.000000000000000000, -1.000000000000000000 ) ) ;
#12044=CARTESIAN_POINT ( 'NONE',  ( 610.0000000000000000, 0.000000000000000000, 210.0000000000000000 ) ) ;
#12056=EDGE_CURVE ( 'NONE', #11914, #9303, #5959, .T. ) ;
#12058=CARTESIAN_POINT ( 'NONE',  ( 10.00000000000000000, 0.000000000000000000, 210.0000000000000000 ) ) ;
#12060=EDGE_LOOP ( 'NONE', ( #5326, #84, #11416, #9004 ) ) ;
#12062=LINE ( 'NONE', #10814, #7113 ) ;
#12064=CARTESIAN_POINT ( 'NONE',  ( 633.0368908673054875, 167.3047950750124642, 210.0000119999999981 ) ) ;
#12070=DIRECTION ( 'NONE',  ( -0.9578262852211508749, 0.2873478855663467724, -0.000000000000000000 ) ) ;
#12080=DIRECTION ( 'NONE',  ( -1.000000000000000000, 0.000000000000000000, 0.000000000000000000 ) ) ;
#12081=MECHANICAL_DESIGN_GEOMETRIC_PRESENTATION_REPRESENTATION('',(#2898),#7366);
#12090=ORIENTED_EDGE ( 'NONE', *, *, #11063, .F. ) ;
#12093=VECTOR ( 'NONE', #8288, 1000.000000000000000 ) ;
#12096=CARTESIAN_POINT ( 'NONE',  ( 10.00000000000000000, -10.00000000000000000, -210.0020000000000095 ) ) ;
#12105=ORIENTED_EDGE ( 'NONE', *, *, #7397, .T. ) ;
#12119=ORIENTED_EDGE ( 'NONE', *, *, #6301, .T. ) ;
#12122=ORIENTED_EDGE ( 'NONE', *, *, #10090, .F. ) ;
#12123=CARTESIAN_POINT ( 'NONE',  ( 635.0000000000000000, 160.0000000000000284, -207.0000000000000000 ) ) ;
#12134=CARTESIAN_POINT ( 'NONE',  ( 139.8040310085880833, 355.9707293956415697, -210.0000000000000000 ) ) ;
#12142=EDGE_CURVE ( 'NONE', #11914, #6340, #7653, .T. ) ;
#12151=EDGE_CURVE ( 'NONE', #12303, #13614, #2185, .T. ) ;
#12154=LINE ( 'NONE', #4195, #5864 ) ;
#12159=ADVANCED_FACE ( 'NONE', ( #4393 ), #6535, .F. ) ;
#12161=DIRECTION ( 'NONE',  ( -1.000000000000000000, 0.000000000000000000, 0.000000000000000000 ) ) ;
#12187=LINE ( 'NONE', #13248, #3821 ) ;
#12193=CARTESIAN_POINT ( 'NONE',  ( 635.0000000000000000, 160.0000000000000284, -207.0000000000000000 ) ) ;
#12199=ORIENTED_EDGE ( 'NONE', *, *, #5984, .T. ) ;
#12203=DIRECTION ( 'NONE',  ( -0.2873478855663453846, -0.9578262852211513190, 0.000000000000000000 ) ) ;
#12218=EDGE_LOOP ( 'NONE', ( #14418, #3614, #13759, #11901 ) ) ;
#12219=AXIS2_PLACEMENT_3D ( 'NONE', #10431, #7106, #4899 ) ;
#12229=CYLINDRICAL_SURFACE ( 'NONE', #10158, 4.199999999999981526 ) ;
#12231=AXIS2_PLACEMENT_3D ( 'NONE', #8984, #3442, #6758 ) ;
#12236=DIRECTION ( 'NONE',  ( 0.2873478855663446629, 0.9578262852211516520, 2.259726690317875391E-15 ) ) ;
#12240=EDGE_CURVE ( 'NONE', #3170, #5923, #6820, .T. ) ;
#12241=EDGE_CURVE ( 'NONE', #5634, #8790, #4619, .T. ) ;
#12244=ORIENTED_EDGE ( 'NONE', *, *, #10461, .T. ) ;
#12246=LINE ( 'NONE', #3553, #8967 ) ;
#12253=VECTOR ( 'NONE', #12632, 1000.000000000000000 ) ;
#12257=AXIS2_PLACEMENT_3D ( 'NONE', #13380, #3143, #4384 ) ;
#12262=ORIENTED_EDGE ( 'NONE', *, *, #10954, .T. ) ;
#12263=EDGE_LOOP ( 'NONE', ( #13652, #1111, #4844, #13613 ) ) ;
#12274=CARTESIAN_POINT ( 'NONE',  ( 635.0000000000000000, 160.0000000000000284, 207.0000000000000000 ) ) ;
#12289=ADVANCED_FACE ( 'NONE', ( #10288 ), #13689, .F. ) ;
#12293=ORIENTED_EDGE ( 'NONE', *, *, #8891, .F. ) ;
#12302=ORIENTED_EDGE ( 'NONE', *, *, #4776, .T. ) ;
#12303=VERTEX_POINT ( 'NONE', #8363 ) ;
#12307=AXIS2_PLACEMENT_3D ( 'NONE', #10599, #12742, #4928 ) ;
#12308=CARTESIAN_POINT ( 'NONE',  ( 633.0483056743199768, 167.3094156464216269, -210.0000000000000284 ) ) ;
#12311=EDGE_CURVE ( 'NONE', #1544, #2949, #459, .T. ) ;
#12318=CARTESIAN_POINT ( 'NONE',  ( 451.6722694765949768, 316.6998517015743460, -210.0000000000000000 ) ) ;
#12330=CARTESIAN_POINT ( 'NONE',  ( 635.0000000000000000, 160.0000000000000284, 207.0000000000000000 ) ) ;
#12331=ORIENTED_EDGE ( 'NONE', *, *, #10835, .F. ) ;
#12332=EDGE_CURVE ( 'NONE', #214, #7052, #7257, .T. ) ;
#12334=ORIENTED_EDGE ( 'NONE', *, *, #10660, .T. ) ;
#12342=ORIENTED_EDGE ( 'NONE', *, *, #13536, .T. ) ;
#12348=LINE ( 'NONE', #13604, #8089 ) ;
#12355=CARTESIAN_POINT ( 'NONE',  ( 148.9991633467111569, 386.6211705227183870, 210.0000000000000000 ) ) ;
#12371=DIRECTION ( 'NONE',  ( -0.000000000000000000, 1.000000000000000000, -0.000000000000000000 ) ) ;
#12374=AXIS2_PLACEMENT_3D ( 'NONE', #1707, #3922, #7168 ) ;
#12402=CARTESIAN_POINT ( 'NONE',  ( 451.6722694765949768, 316.6998517015743460, -190.0000000000000000 ) ) ;
#12412=AXIS2_PLACEMENT_3D ( 'NONE', #11143, #12236, #8636 ) ;
#12416=DIRECTION ( 'NONE',  ( 1.000000000000000000, 0.000000000000000000, 0.000000000000000000 ) ) ;
#12419=CARTESIAN_POINT ( 'NONE',  ( 650.0000000000000000, 145.0000000000000568, 210.0000000000000000 ) ) ;
#12420=EDGE_LOOP ( 'NONE', ( #12808, #3436, #13716, #8749 ) ) ;
#12421=CYLINDRICAL_SURFACE ( 'NONE', #9434, 4.199999999999981526 ) ;
#12426=ADVANCED_FACE ( 'NONE', ( #6293 ), #674, .T. ) ;
#12428=AXIS2_PLACEMENT_3D ( 'NONE', #12419, #6896, #5507 ) ;
#12430=DIRECTION ( 'NONE',  ( 0.000000000000000000, 0.000000000000000000, 1.000000000000000000 ) ) ;
#12431=FACE_OUTER_BOUND ( 'NONE', #6833, .T. ) ;
#12434=PLANE ( 'NONE',  #12231 ) ;
#12438=FACE_OUTER_BOUND ( 'NONE', #13293, .T. ) ;
#12441=LINE ( 'NONE', #7885, #2582 ) ;
#12442=ORIENTED_EDGE ( 'NONE', *, *, #4089, .T. ) ;
#12455=DIRECTION ( 'NONE',  ( 0.2873478855663453846, 0.9578262852211513190, 0.000000000000000000 ) ) ;
#12468=AXIS2_PLACEMENT_3D ( 'NONE', #4138, #1915, #12015 ) ;
#12472=ORIENTED_EDGE ( 'NONE', *, *, #4100, .T. ) ;
#12475=CARTESIAN_POINT ( 'NONE',  ( 590.0000000000000000, 10.00000000000005507, -210.0020000000000095 ) ) ;
#12479=VERTEX_POINT ( 'NONE', #7413 ) ;
#12484=AXIS2_PLACEMENT_3D ( 'NONE', #6790, #5542, #3338 ) ;
#12505=EDGE_LOOP ( 'NONE', ( #5730, #14523 ) ) ;
#12511=CARTESIAN_POINT ( 'NONE',  ( -9.498873539028489220E-16, 10.00000000000000000, -210.0000000000000000 ) ) ;
#12517=DIRECTION ( 'NONE',  ( 0.000000000000000000, -1.000000000000000000, 0.000000000000000000 ) ) ;
#12518=AXIS2_PLACEMENT_3D ( 'NONE', #7726, #5445, #9947 ) ;
#12523=VERTEX_POINT ( 'NONE', #757 ) ;
#12540=ORIENTED_EDGE ( 'NONE', *, *, #7246, .F. ) ;
#12559=DIRECTION ( 'NONE',  ( -0.9578262852211517631, 0.2873478855663438858, -0.000000000000000000 ) ) ;
#12573=ORIENTED_EDGE ( 'NONE', *, *, #1499, .T. ) ;
#12577=CARTESIAN_POINT ( 'NONE',  ( 640.2500000000000000, 160.0000000000000284, 207.0000000000000000 ) ) ;
#12587=FACE_OUTER_BOUND ( 'NONE', #8048, .T. ) ;
#12592=LINE ( 'NONE', #2476, #11935 ) ;
#12594=ADVANCED_FACE ( 'NONE', ( #3349 ), #10123, .F. ) ;
#12599=ORIENTED_EDGE ( 'NONE', *, *, #498, .T. ) ;
#12605=EDGE_CURVE ( 'NONE', #2635, #7765, #10272, .T. ) ;
#12618=EDGE_LOOP ( 'NONE', ( #5561, #5540, #13123, #414 ) ) ;
#12619=CARTESIAN_POINT ( 'NONE',  ( 610.0000000000000000, -9.999999999999941380, -210.0000000000000000 ) ) ;
#12625=CARTESIAN_POINT ( 'NONE',  ( 9.498873539028489220E-16, -10.00000000000000000, 210.0000000000000000 ) ) ;
#12632=DIRECTION ( 'NONE',  ( 1.000000000000000000, 0.000000000000000000, 0.000000000000000000 ) ) ;
#12634=EDGE_LOOP ( 'NONE', ( #5066, #11187, #932, #7750, #5752, #842, #292, #6753, #11753, #586, #6971, #7221, #5572, #5886, #13894, #2241, #11715, #5270, #2882, #7796 ) ) ;
#12635=CARTESIAN_POINT ( 'NONE',  ( 631.2228576472183477, 153.4466020873430239, 210.0000120000000265 ) ) ;
#12638=ORIENTED_EDGE ( 'NONE', *, *, #9050, .F. ) ;
#12640=CARTESIAN_POINT ( 'NONE',  ( 10.00000000000000000, 10.00000000000000178, -210.0020000000000095 ) ) ;
#12646=EDGE_LOOP ( 'NONE', ( #4621, #1104 ) ) ;
#12653=EDGE_CURVE ( 'NONE', #8972, #1538, #10206, .T. ) ;
#12656=CARTESIAN_POINT ( 'NONE',  ( 650.0000000000000000, 175.0000000000000568, -210.0000000000000000 ) ) ;
#12665=VERTEX_POINT ( 'NONE', #13368 ) ;
#12668=CARTESIAN_POINT ( 'NONE',  ( 145.1678582058265476, 408.6511750828048548, 190.0000000000000000 ) ) ;
#12669=EDGE_CURVE ( 'NONE', #14275, #14524, #974, .T. ) ;
#12687=AXIS2_PLACEMENT_3D ( 'NONE', #5506, #3148, #1055 ) ;
#12688=ORIENTED_EDGE ( 'NONE', *, *, #3396, .T. ) ;
#12691=DIRECTION ( 'NONE',  ( -0.000000000000000000, -0.000000000000000000, -1.000000000000000000 ) ) ;
#12693=PLANE ( 'NONE',  #5909 ) ;
#12706=EDGE_CURVE ( 'NONE', #11363, #14510, #13889, .T. ) ;
#12707=ORIENTED_EDGE ( 'NONE', *, *, #13561, .T. ) ;
#12711=AXIS2_PLACEMENT_3D ( 'NONE', #589, #528, #4154 ) ;
#12719=VECTOR ( 'NONE', #2100, 1000.000000000000000 ) ;
#12720=AXIS2_PLACEMENT_3D ( 'NONE', #2390, #13318, #4389 ) ;
#12722=PLANE ( 'NONE',  #11487 ) ;
#12728=VECTOR ( 'NONE', #8742, 1000.000000000000114 ) ;
#12740=AXIS2_PLACEMENT_3D ( 'NONE', #134, #3417, #9026 ) ;
#12742=DIRECTION ( 'NONE',  ( -0.2873478855663454401, -0.9578262852211514300, 0.000000000000000000 ) ) ;
#12750=ADVANCED_FACE ( 'NONE', ( #11660, #7236, #10488, #1553, #11517, #10341, #12923 ), #7095, .T. ) ;
#12758=DIRECTION ( 'NONE',  ( 1.000000000000000000, 0.000000000000000000, 0.000000000000000000 ) ) ;
#12769=EDGE_LOOP ( 'NONE', ( #10821, #8415, #12119, #3171 ) ) ;
#12775=PRODUCT_DEFINITION_SHAPE ( 'NONE', 'NONE',  #6844 ) ;
#12808=ORIENTED_EDGE ( 'NONE', *, *, #5160, .F. ) ;
#12810=AXIS2_PLACEMENT_3D ( 'NONE', #1211, #3367, #14571 ) ;
#12811=DIRECTION ( 'NONE',  ( -0.2873478855663453846, -0.9578262852211513190, -0.000000000000000000 ) ) ;
#12814=PLANE ( 'NONE',  #7965 ) ;
#12817=CARTESIAN_POINT ( 'NONE',  ( 145.1678582058265192, 408.6511750828049117, 210.0000000000000000 ) ) ;
#12819=FACE_OUTER_BOUND ( 'NONE', #8558, .T. ) ;
#12825=CARTESIAN_POINT ( 'NONE',  ( 451.6722694765949768, 316.6998517015743460, -210.0000000000000000 ) ) ;
#12827=CARTESIAN_POINT ( 'NONE',  ( 635.0000000000000000, 160.0000000000000284, 190.0000000000000284 ) ) ;
#12836=ORIENTED_EDGE ( 'NONE', *, *, #11803, .F. ) ;
#12837=CARTESIAN_POINT ( 'NONE',  ( 10.00000000000000000, 10.00000000000000178, -190.0000000000000000 ) ) ;
#12838=CARTESIAN_POINT ( 'NONE',  ( 133.6739427831727198, 370.3381236739588758, 210.0000000000000000 ) ) ;
#12863=ORIENTED_EDGE ( 'NONE', *, *, #7139, .F. ) ;
#12865=DIRECTION ( 'NONE',  ( -1.000000000000000000, -0.000000000000000000, -0.000000000000000000 ) ) ;
#12868=DIRECTION ( 'NONE',  ( 0.000000000000000000, 0.000000000000000000, -1.000000000000000000 ) ) ;
#12876=ORIENTED_EDGE ( 'NONE', *, *, #11158, .T. ) ;
#12878=EDGE_CURVE ( 'NONE', #9599, #1319, #7532, .T. ) ;
#12879=FACE_OUTER_BOUND ( 'NONE', #7261, .T. ) ;
#12881=CYLINDRICAL_SURFACE ( 'NONE', #2538, 7.500000000000062172 ) ;
#12885=LINE ( 'NONE', #14009, #5369 ) ;
#12895=PRODUCT ( 'main frame', 'main frame', '', ( #10033 ) ) ;
#12896=DIRECTION ( 'NONE',  ( 0.000000000000000000, 1.000000000000000000, 0.000000000000000000 ) ) ;
#12898=VERTEX_POINT ( 'NONE', #13003 ) ;
#12899=CARTESIAN_POINT ( 'NONE',  ( 145.1678582058265192, 408.6511750828049117, -210.0000000000000000 ) ) ;
#12902=DIRECTION ( 'NONE',  ( -0.000000000000000000, -0.000000000000000000, 1.000000000000000000 ) ) ;
#12905=VERTEX_POINT ( 'NONE', #5106 ) ;
#12917=B_SPLINE_CURVE_WITH_KNOTS ( 'NONE', 3,
 ( #6243, #11911, #2928, #6313, #10742, #613, #2992, #5139, #10815, #7489, #12064, #691, #9720, #1958, #14220, #6469, #4114, #7649 ),
 .UNSPECIFIED., .F., .F.,
 ( 4, 2, 2, 2, 2, 2, 2, 2, 4 ),
 ( 0.000000000000000000, 0.06250000000000000000, 0.1250000000000000000, 0.1875000000000000000, 0.2500000000000000000, 0.3125000000000000000, 0.3750000000000000000, 0.4375000000000000000, 0.5000000000000000000 ),
 .UNSPECIFIED. ) ;
#12923=FACE_BOUND ( 'NONE', #12646, .T. ) ;
#12925=DIRECTION ( 'NONE',  ( -1.000000000000000000, 0.000000000000000000, 0.000000000000000000 ) ) ;
#12927=ORIENTED_EDGE ( 'NONE', *, *, #5341, .T. ) ;
#12930=EDGE_CURVE ( 'NONE', #7999, #2271, #9601, .T. ) ;
#12947=VERTEX_POINT ( 'NONE', #5323 ) ;
#12948=EDGE_LOOP ( 'NONE', ( #14153, #7856, #5915, #3570, #2157, #4277, #1970, #11124 ) ) ;
#12953=DIRECTION ( 'NONE',  ( -1.000000000000000000, 0.000000000000000000, 0.000000000000000000 ) ) ;
#12954=VECTOR ( 'NONE', #6447, 1000.000000000000000 ) ;
#12961=DIRECTION ( 'NONE',  ( 0.000000000000000000, 1.000000000000000000, 0.000000000000000000 ) ) ;
#12966=CARTESIAN_POINT ( 'NONE',  ( 10.00000000000000000, 0.000000000000000000, -190.0000000000000000 ) ) ;
#12976=CARTESIAN_POINT ( 'NONE',  ( -9.498873539028489220E-16, 10.00000000000000000, -190.0000000000000000 ) ) ;
#12979=VECTOR ( 'NONE', #8290, 1000.000000000000114 ) ;
#12994=CARTESIAN_POINT ( 'NONE',  ( 139.8040310085880833, 355.9707293956415697, 187.0000000000000000 ) ) ;
#12997=CARTESIAN_POINT ( 'NONE',  ( 650.0000000000000000, 175.0000000000000568, 210.0000000000000000 ) ) ;
#13000=ORIENTED_EDGE ( 'NONE', *, *, #3960, .F. ) ;
#13003=CARTESIAN_POINT ( 'NONE',  ( 640.2500000000000000, 160.0000000000000284, -207.0000000000000000 ) ) ;
#13009=AXIS2_PLACEMENT_3D ( 'NONE', #13707, #5797, #3520 ) ;
#13010=FACE_OUTER_BOUND ( 'NONE', #4929, .T. ) ;
#13013=FACE_OUTER_BOUND ( 'NONE', #3486, .T. ) ;
#13028=PRODUCT_DEFINITION_FORMATION_WITH_SPECIFIED_SOURCE ( 'ANY', '', #12895, .NOT_KNOWN. ) ;
#13034=VECTOR ( 'NONE', #13448, 1000.000000000000000 ) ;
#13041=EDGE_CURVE ( 'NONE', #14011, #9542, #6651, .T. ) ;
#13044=DIRECTION ( 'NONE',  ( -1.000000000000000000, -0.000000000000000000, -0.000000000000000000 ) ) ;
#13046=VECTOR ( 'NONE', #1884, 1000.000000000000000 ) ;
#13075=CARTESIAN_POINT ( 'NONE',  ( 451.6722694765949768, 316.6998517015743460, 210.0000000000000000 ) ) ;
#13079=ADVANCED_FACE ( 'NONE', ( #1027 ), #619, .F. ) ;
#13083=DIRECTION ( 'NONE',  ( -0.000000000000000000, -0.000000000000000000, -1.000000000000000000 ) ) ;
#13084=CARTESIAN_POINT ( 'NONE',  ( 112.9652219749295341, 376.5507399164317803, 210.0000000000000000 ) ) ;
#13091=DIRECTION ( 'NONE',  ( 0.000000000000000000, 0.000000000000000000, -1.000000000000000000 ) ) ;
#13100=LINE ( 'NONE', #4242, #12728 ) ;
#13101=DIRECTION ( 'NONE',  ( -0.000000000000000000, -0.000000000000000000, -1.000000000000000000 ) ) ;
#13103=EDGE_LOOP ( 'NONE', ( #2395, #1195, #6892, #9728 ) ) ;
#13104=CARTESIAN_POINT ( 'NONE',  ( 448.9584422793565750, 264.0194060144110608, -190.0000000000000000 ) ) ;
#13106=CARTESIAN_POINT ( 'NONE',  ( 145.1678582058265192, 408.6511750828049117, -210.0000000000000000 ) ) ;
#13112=EDGE_LOOP ( 'NONE', ( #8069, #11316, #770, #3311 ) ) ;
#13114=VERTEX_POINT ( 'NONE', #9649 ) ;
#13120=CARTESIAN_POINT ( 'NONE',  ( 455.5035746174796714, 294.6698471414878782, -210.0000000000000000 ) ) ;
#13123=ORIENTED_EDGE ( 'NONE', *, *, #4950, .F. ) ;
#13127=EDGE_LOOP ( 'NONE', ( #9783, #9296, #14018, #11760 ) ) ;
#13133=VECTOR ( 'NONE', #7811, 1000.000000000000000 ) ;
#13135=DIRECTION ( 'NONE',  ( -0.000000000000000000, -0.000000000000000000, -1.000000000000000000 ) ) ;
#13144=LINE ( 'NONE', #13221, #12024 ) ;
#13145=CIRCLE ( 'NONE', #14095, 2.649999999999985700 ) ;
#13146=ORIENTED_EDGE ( 'NONE', *, *, #7541, .T. ) ;
#13149=CARTESIAN_POINT ( 'NONE',  ( 610.0000000000000000, 10.00000000000005507, -210.0020000000000095 ) ) ;
#13158=EDGE_CURVE ( 'NONE', #2989, #7099, #14074, .T. ) ;
#13184=CARTESIAN_POINT ( 'NONE',  ( 164.3243839102495656, 402.9042173714779551, -210.0000000000000000 ) ) ;
#13190=EDGE_LOOP ( 'NONE', ( #476, #3886 ) ) ;
#13195=SURFACE_SIDE_STYLE ('',( #13275 ) ) ;
#13204=EDGE_LOOP ( 'NONE', ( #7030, #5332, #7918, #4949 ) ) ;
#13208=PLANE ( 'NONE',  #929 ) ;
#13209=DIRECTION ( 'NONE',  ( 0.000000000000000000, -1.000000000000000000, 0.000000000000000000 ) ) ;
#13210=COLOUR_RGB ( '',0.8941176470588234615, 0.8941176470588234615, 0.8941176470588234615 ) ;
#13213=DIRECTION ( 'NONE',  ( -1.000000000000000000, 0.000000000000000000, 0.000000000000000000 ) ) ;
#13214=ADVANCED_FACE ( 'NONE', ( #1889 ), #779, .F. ) ;
#13220=AXIS2_PLACEMENT_3D ( 'NONE', #10927, #14097, #799 ) ;
#13221=CARTESIAN_POINT ( 'NONE',  ( 145.1678582058265192, 408.6511750828049117, -210.0000000000000000 ) ) ;
#13222=ORIENTED_EDGE ( 'NONE', *, *, #5745, .F. ) ;
#13230=DIRECTION ( 'NONE',  ( -0.000000000000000000, -0.000000000000000000, -1.000000000000000000 ) ) ;
#13241=AXIS2_PLACEMENT_3D ( 'NONE', #2032, #6547, #2940 ) ;
#13243=AXIS2_PLACEMENT_3D ( 'NONE', #12123, #4168, #5204 ) ;
#13248=CARTESIAN_POINT ( 'NONE',  ( 10.00000000000000000, 0.000000000000000000, -210.0000000000000000 ) ) ;
#13274=PLANE ( 'NONE',  #14216 ) ;
#13275=SURFACE_STYLE_FILL_AREA ( #5242 ) ;
#13282=CARTESIAN_POINT ( 'NONE',  ( 627.5000000000000000, 159.0056981173382553, -209.9999999999999716 ) ) ;
#13291=CARTESIAN_POINT ( 'NONE',  ( 610.0000000000000000, 0.000000000000000000, 210.0000000000000000 ) ) ;
#13293=EDGE_LOOP ( 'NONE', ( #11643, #10020, #12331, #11765 ) ) ;
#13303=PLANE ( 'NONE',  #3513 ) ;
#13315=ORIENTED_EDGE ( 'NONE', *, *, #6573, .F. ) ;
#13318=DIRECTION ( 'NONE',  ( -9.498873539028489960E-17, 1.000000000000000000, 0.000000000000000000 ) ) ;
#13323=ORIENTED_EDGE ( 'NONE', *, *, #5920, .T. ) ;
#13346=CARTESIAN_POINT ( 'NONE',  ( 635.0000000000000000, 160.0000000000000284, 207.0000000000000000 ) ) ;
#13361=DIRECTION ( 'NONE',  ( 1.000000000000000000, 0.000000000000000000, 0.000000000000000000 ) ) ;
#13368=CARTESIAN_POINT ( 'NONE',  ( 10.00000000000000000, -9.999999999999998224, 190.0000000000000000 ) ) ;
#13371=ADVANCED_FACE ( 'NONE', ( #5054 ), #5269, .F. ) ;
#13380=CARTESIAN_POINT ( 'NONE',  ( 446.3084422793565409, 264.0194060144110608, 187.0000000000000000 ) ) ;
#13390=EDGE_CURVE ( 'NONE', #6556, #9876, #848, .T. ) ;
#13392=AXIS2_PLACEMENT_3D ( 'NONE', #3021, #9454, #725 ) ;
#13396=VERTEX_POINT ( 'NONE', #713 ) ;
#13398=ORIENTED_EDGE ( 'NONE', *, *, #14083, .T. ) ;
#13420=CARTESIAN_POINT ( 'NONE',  ( 627.5000000000000000, 160.0000000000000284, -210.0000059999999849 ) ) ;
#13424=VECTOR ( 'NONE', #12896, 1000.000000000000000 ) ;
#13448=DIRECTION ( 'NONE',  ( -0.000000000000000000, -0.000000000000000000, -1.000000000000000000 ) ) ;
#13449=ORIENTED_EDGE ( 'NONE', *, *, #14225, .F. ) ;
#13450=AXIS2_PLACEMENT_3D ( 'NONE', #6973, #4627, #244 ) ;
#13453=CARTESIAN_POINT ( 'NONE',  ( 610.0000000000000000, 227.4403065089105951, 210.0000000000000000 ) ) ;
#13456=FACE_OUTER_BOUND ( 'NONE', #13204, .T. ) ;
#13478=ORIENTED_EDGE ( 'NONE', *, *, #4575, .T. ) ;
#13485=FACE_OUTER_BOUND ( 'NONE', #7903, .T. ) ;
#13489=CARTESIAN_POINT ( 'NONE',  ( 650.0000000000000000, 175.0000000000000568, 190.0000000000000000 ) ) ;
#13491=CARTESIAN_POINT ( 'NONE',  ( 650.0000000000000000, 145.0000000000000568, 210.0000000000000000 ) ) ;
#13499=CARTESIAN_POINT ( 'NONE',  ( 112.9652219749295341, 376.5507399164317803, 190.0000000000000000 ) ) ;
#13509=PLANE ( 'NONE',  #3652 ) ;
#13521=CARTESIAN_POINT ( 'NONE',  ( 455.5035746174796714, 294.6698471414878782, 210.0000000000000000 ) ) ;
#13533=ORIENTED_EDGE ( 'NONE', *, *, #6792, .T. ) ;
#13536=EDGE_CURVE ( 'NONE', #10228, #10517, #1156, .T. ) ;
#13561=EDGE_CURVE ( 'NONE', #13629, #7886, #2099, .T. ) ;
#13566=CARTESIAN_POINT ( 'NONE',  ( 470.8287951810180516, 310.9528939902474463, 210.0000000000000000 ) ) ;
#13577=EDGE_CURVE ( 'NONE', #8790, #3368, #5659, .T. ) ;
#13583=ADVANCED_FACE ( 'NONE', ( #2411 ), #12434, .F. ) ;
#13584=CARTESIAN_POINT ( 'NONE',  ( 610.0000000000000000, 0.000000000000000000, 210.0000000000000000 ) ) ;
#13586=LINE ( 'NONE', #283, #489 ) ;
#13603=VECTOR ( 'NONE', #1227, 1000.000000000000114 ) ;
#13604=CARTESIAN_POINT ( 'NONE',  ( 112.9652219749295341, 376.5507399164317803, -190.0000000000000000 ) ) ;
#13606=LINE ( 'NONE', #14569, #9194 ) ;
#13609=DIRECTION ( 'NONE',  ( -0.000000000000000000, -0.000000000000000000, 1.000000000000000000 ) ) ;
#13613=ORIENTED_EDGE ( 'NONE', *, *, #12311, .F. ) ;
#13614=VERTEX_POINT ( 'NONE', #7941 ) ;
#13620=CARTESIAN_POINT ( 'NONE',  ( 153.1991633467111456, 386.6211705227183870, 190.0000000000000000 ) ) ;
#13629=VERTEX_POINT ( 'NONE', #10299 ) ;
#13638=FACE_OUTER_BOUND ( 'NONE', #14581, .T. ) ;
#13652=ORIENTED_EDGE ( 'NONE', *, *, #7541, .F. ) ;
#13661=EDGE_CURVE ( 'NONE', #6556, #5961, #9120, .T. ) ;
#13665=VECTOR ( 'NONE', #10069, 1000.000000000000114 ) ;
#13670=DIRECTION ( 'NONE',  ( -0.000000000000000000, -0.000000000000000000, -1.000000000000000000 ) ) ;
#13676=CARTESIAN_POINT ( 'NONE',  ( 590.0000000000000000, -9.999999999999941380, -210.0020000000000095 ) ) ;
#13677=CIRCLE ( 'NONE', #466, 2.649999999999985700 ) ;
#13689=CYLINDRICAL_SURFACE ( 'NONE', #12810, 4.199999999999981526 ) ;
#13693=AXIS2_PLACEMENT_3D ( 'NONE', #656, #8574, #5108 ) ;
#13703=VECTOR ( 'NONE', #9950, 1000.000000000000114 ) ;
#13706=ORIENTED_EDGE ( 'NONE', *, *, #10896, .F. ) ;
#13707=CARTESIAN_POINT ( 'NONE',  ( 650.0000000000000000, 0.000000000000000000, 0.000000000000000000 ) ) ;
#13713=ORIENTED_EDGE ( 'NONE', *, *, #7513, .T. ) ;
#13716=ORIENTED_EDGE ( 'NONE', *, *, #8065, .F. ) ;
#13721=DIRECTION ( 'NONE',  ( -0.000000000000000000, 1.000000000000000000, -0.000000000000000000 ) ) ;
#13728=CARTESIAN_POINT ( 'NONE',  ( 153.1991633467111456, 386.6211705227183870, -210.0000000000000000 ) ) ;
#13743=CARTESIAN_POINT ( 'NONE',  ( 112.9652219749295341, 376.5507399164317803, -210.0000000000000000 ) ) ;
#13749=DIRECTION ( 'NONE',  ( 1.000000000000000000, 0.000000000000000000, -0.000000000000000000 ) ) ;
#13751=LINE ( 'NONE', #3644, #12253 ) ;
#13754=DIRECTION ( 'NONE',  ( -0.000000000000000000, -0.000000000000000000, -1.000000000000000000 ) ) ;
#13759=ORIENTED_EDGE ( 'NONE', *, *, #9050, .T. ) ;
#13766=ORIENTED_EDGE ( 'NONE', *, *, #13390, .F. ) ;
#13768=ORIENTED_EDGE ( 'NONE', *, *, #10260, .F. ) ;
#13772=ADVANCED_FACE ( 'NONE', ( #7203 ), #6978, .F. ) ;
#13773=PLANE ( 'NONE',  #13450 ) ;
#13775=DIRECTION ( 'NONE',  ( 0.000000000000000000, 0.000000000000000000, -1.000000000000000000 ) ) ;
#13789=DIRECTION ( 'NONE',  ( -0.2873478855663453846, -0.9578262852211513190, -0.000000000000000000 ) ) ;
#13793=EDGE_LOOP ( 'NONE', ( #7157, #5584, #14426, #620 ) ) ;
#13819=LINE ( 'NONE', #1496, #7722 ) ;
#13825=EDGE_CURVE ( 'NONE', #9797, #4375, #387, .T. ) ;
#13839=LINE ( 'NONE', #6307, #11717 ) ;
#13840=ORIENTED_EDGE ( 'NONE', *, *, #1647, .F. ) ;
#13849=VECTOR ( 'NONE', #3657, 1000.000000000000000 ) ;
#13852=VECTOR ( 'NONE', #12559, 1000.000000000000227 ) ;
#13868=VERTEX_POINT ( 'NONE', #9639 ) ;
#13872=DIRECTION ( 'NONE',  ( -0.000000000000000000, -0.000000000000000000, -1.000000000000000000 ) ) ;
#13887=ORIENTED_EDGE ( 'NONE', *, *, #9085, .T. ) ;
#13889=LINE ( 'NONE', #2597, #6327 ) ;
#13894=ORIENTED_EDGE ( 'NONE', *, *, #5655, .T. ) ;
#13898=AXIS2_PLACEMENT_3D ( 'NONE', #13120, #9800, #8901 ) ;
#13901=VERTEX_POINT ( 'NONE', #7351 ) ;
#13902=EDGE_CURVE ( 'NONE', #10585, #8377, #8530, .T. ) ;
#13909=DIRECTION ( 'NONE',  ( -0.000000000000000000, -0.000000000000000000, 1.000000000000000000 ) ) ;
#13922=EDGE_CURVE ( 'NONE', #14108, #10070, #12917, .T. ) ;
#13924=VECTOR ( 'NONE', #14087, 1000.000000000000000 ) ;
#13927=AXIS2_PLACEMENT_3D ( 'NONE', #12330, #13230, #13361 ) ;
#13939=DIRECTION ( 'NONE',  ( -1.000000000000000000, 0.000000000000000000, 0.000000000000000000 ) ) ;
#13942=DIRECTION ( 'NONE',  ( 1.000000000000000000, 0.000000000000000000, 0.000000000000000000 ) ) ;
#13951=ORIENTED_EDGE ( 'NONE', *, *, #1146, .F. ) ;
#13963=B_SPLINE_CURVE_WITH_KNOTS ( 'NONE', 3,
 ( #5995, #5775, #6885, #4829, #3572, #1277, #12635, #9168, #10348, #8127, #10278, #9322, #4897, #216, #137, #444, #4763, #9392 ),
 .UNSPECIFIED., .F., .F.,
 ( 4, 2, 2, 2, 2, 2, 2, 2, 4 ),
 ( 0.5000000000000000000, 0.5625000000000000000, 0.6250000000000000000, 0.6875000000000000000, 0.7500000000000000000, 0.8125000000000000000, 0.8750000000000000000, 0.9375000000000000000, 1.000000000000000000 ),
 .UNSPECIFIED. ) ;
#13965=DIRECTION ( 'NONE',  ( -9.498873539028489960E-17, 1.000000000000000000, 0.000000000000000000 ) ) ;
#13970=ORIENTED_EDGE ( 'NONE', *, *, #2759, .T. ) ;
#13977=ORIENTED_EDGE ( 'NONE', *, *, #472, .F. ) ;
#13983=AXIS2_PLACEMENT_3D ( 'NONE', #9122, #2477, #3523 ) ;
#13985=EDGE_CURVE ( 'NONE', #3336, #12479, #3209, .T. ) ;
#13996=ORIENTED_EDGE ( 'NONE', *, *, #6432, .T. ) ;
#13999=ORIENTED_EDGE ( 'NONE', *, *, #12669, .F. ) ;
#14009=CARTESIAN_POINT ( 'NONE',  ( 610.0000000000000000, 0.000000000000000000, -190.0000000000000000 ) ) ;
#14011=VERTEX_POINT ( 'NONE', #76 ) ;
#14014=VERTEX_POINT ( 'NONE', #1123 ) ;
#14018=ORIENTED_EDGE ( 'NONE', *, *, #1975, .F. ) ;
#14036=CARTESIAN_POINT ( 'NONE',  ( 142.4540310085880606, 355.9707293956415697, -190.0000000000000000 ) ) ;
#14037=EDGE_CURVE ( 'NONE', #9599, #14014, #13606, .T. ) ;
#14055=CARTESIAN_POINT ( 'NONE',  ( 459.3348797583642522, 272.6398425814014104, 210.0000000000000000 ) ) ;
#14056=CARTESIAN_POINT ( 'NONE',  ( 164.3243839102495656, 402.9042173714779551, 190.0000000000000000 ) ) ;
#14063=EDGE_CURVE ( 'NONE', #5539, #793, #10127, .T. ) ;
#14064=ADVANCED_FACE ( 'NONE', ( #6682 ), #2301, .T. ) ;
#14065=CARTESIAN_POINT ( 'NONE',  ( 470.8287951810180516, 310.9528939902474463, -190.0000000000000000 ) ) ;
#14069=CARTESIAN_POINT ( 'NONE',  ( 448.9584422793565750, 264.0194060144110608, -210.0000000000000000 ) ) ;
#14074=LINE ( 'NONE', #12966, #7517 ) ;
#14077=CARTESIAN_POINT ( 'NONE',  ( 446.3084422793565409, 264.0194060144110608, -210.0000000000000000 ) ) ;
#14080=ORIENTED_EDGE ( 'NONE', *, *, #5409, .T. ) ;
#14083=EDGE_CURVE ( 'NONE', #13629, #5518, #7710, .T. ) ;
#14086=( NAMED_UNIT ( * ) PLANE_ANGLE_UNIT ( ) SI_UNIT ( $, .RADIAN. ) );
#14087=DIRECTION ( 'NONE',  ( 0.000000000000000000, 0.000000000000000000, -1.000000000000000000 ) ) ;
#14091=ORIENTED_EDGE ( 'NONE', *, *, #3511, .T. ) ;
#14092=VERTEX_POINT ( 'NONE', #10062 ) ;
#14095=AXIS2_PLACEMENT_3D ( 'NONE', #2237, #10221, #6745 ) ;
#14097=DIRECTION ( 'NONE',  ( -0.000000000000000000, -0.000000000000000000, 1.000000000000000000 ) ) ;
#14108=VERTEX_POINT ( 'NONE', #6743 ) ;
#14113=EDGE_CURVE ( 'NONE', #6071, #11023, #11242, .T. ) ;
#14118=CARTESIAN_POINT ( 'NONE',  ( 10.00000000000000000, 10.00000000000000178, -210.0000000000000000 ) ) ;
#14122=DIRECTION ( 'NONE',  ( -0.000000000000000000, -0.000000000000000000, -1.000000000000000000 ) ) ;
#14124=CARTESIAN_POINT ( 'NONE',  ( 590.0000000000000000, 0.000000000000000000, 210.0000000000000000 ) ) ;
#14135=DIRECTION ( 'NONE',  ( 0.000000000000000000, 0.000000000000000000, 1.000000000000000000 ) ) ;
#14140=EDGE_LOOP ( 'NONE', ( #6733, #8889 ) ) ;
#14145=EDGE_CURVE ( 'NONE', #9301, #6798, #1566, .T. ) ;
#14153=ORIENTED_EDGE ( 'NONE', *, *, #2207, .T. ) ;
#14179=CARTESIAN_POINT ( 'NONE',  ( 641.0061384268468601, 164.6003227093606540, -210.0000000000000000 ) ) ;
#14189=FACE_OUTER_BOUND ( 'NONE', #7806, .T. ) ;
#14193=CARTESIAN_POINT ( 'NONE',  ( 635.0000000000000000, 160.0000000000000284, -210.0000000000000000 ) ) ;
#14198=ORIENTED_EDGE ( 'NONE', *, *, #5498, .T. ) ;
#14200=CARTESIAN_POINT ( 'NONE',  ( 137.1540310085880776, 355.9707293956415697, -190.0000000000000000 ) ) ;
#14216=AXIS2_PLACEMENT_3D ( 'NONE', #14301, #1903, #1009 ) ;
#14219=ORIENTED_EDGE ( 'NONE', *, *, #3968, .T. ) ;
#14220=CARTESIAN_POINT ( 'NONE',  ( 628.4466020873430807, 163.7771423527818229, 210.0000119999999981 ) ) ;
#14221=CARTESIAN_POINT ( 'NONE',  ( 451.6722694765949768, 316.6998517015743460, 210.0000000000000000 ) ) ;
#14225=EDGE_CURVE ( 'NONE', #12905, #9276, #4985, .T. ) ;
#14241=VERTEX_POINT ( 'NONE', #5272 ) ;
#14242=CARTESIAN_POINT ( 'NONE',  ( 145.1678582058265192, 408.6511750828049117, 210.0000000000000000 ) ) ;
#14251=EDGE_CURVE ( 'NONE', #6798, #6803, #14269, .T. ) ;
#14269=LINE ( 'NONE', #6227, #7314 ) ;
#14275=VERTEX_POINT ( 'NONE', #10794 ) ;
#14285=DIRECTION ( 'NONE',  ( 1.000000000000000000, 0.000000000000000000, 0.000000000000000000 ) ) ;
#14295=DIRECTION ( 'NONE',  ( 0.000000000000000000, 0.000000000000000000, 1.000000000000000000 ) ) ;
#14301=CARTESIAN_POINT ( 'NONE',  ( 635.0000000000000000, 160.0000000000000284, 207.0000000000000000 ) ) ;
#14302=DIRECTION ( 'NONE',  ( 0.000000000000000000, 0.000000000000000000, 1.000000000000000000 ) ) ;
#14310=ADVANCED_FACE ( 'NONE', ( #3322 ), #534, .F. ) ;
#14311=CARTESIAN_POINT ( 'NONE',  ( 642.5000000000001137, 160.0000000000000284, -210.0000059999999849 ) ) ;
#14312=VECTOR ( 'NONE', #11066, 1000.000000000000000 ) ;
#14320=LINE ( 'NONE', #3244, #14312 ) ;
#14323=CIRCLE ( 'NONE', #11477, 4.199999999999981526 ) ;
#14328=EDGE_LOOP ( 'NONE', ( #187, #13315, #14414, #6424 ) ) ;
#14330=CARTESIAN_POINT ( 'NONE',  ( 451.6722694765949768, 316.6998517015743460, -210.0000000000000000 ) ) ;
#14336=VECTOR ( 'NONE', #13909, 1000.000000000000000 ) ;
#14343=CARTESIAN_POINT ( 'NONE',  ( 610.0000000000000000, 145.0000000000000568, -210.0000000000000000 ) ) ;
#14348=AXIS2_PLACEMENT_3D ( 'NONE', #14124, #7556, #10798 ) ;
#14351=LINE ( 'NONE', #8955, #3331 ) ;
#14356=CARTESIAN_POINT ( 'NONE',  ( 153.1991633467111456, 386.6211705227183870, -190.0000000000000000 ) ) ;
#14385=FACE_OUTER_BOUND ( 'NONE', #7530, .T. ) ;
#14386=VECTOR ( 'NONE', #13670, 1000.000000000000000 ) ;
#14392=VECTOR ( 'NONE', #7450, 1000.000000000000000 ) ;
#14394=ORIENTED_EDGE ( 'NONE', *, *, #2775, .F. ) ;
#14401=DIRECTION ( 'NONE',  ( 0.9578262852211517631, -0.2873478855663438858, 0.000000000000000000 ) ) ;
#14402=ORIENTED_EDGE ( 'NONE', *, *, #2310, .T. ) ;
#14410=ADVANCED_FACE ( 'NONE', ( #6992 ), #3621, .T. ) ;
#14413=VECTOR ( 'NONE', #1813, 1000.000000000000000 ) ;
#14414=ORIENTED_EDGE ( 'NONE', *, *, #3686, .T. ) ;
#14418=ORIENTED_EDGE ( 'NONE', *, *, #5456, .T. ) ;
#14426=ORIENTED_EDGE ( 'NONE', *, *, #3396, .F. ) ;
#14428=APPLICATION_CONTEXT ( 'automotive_design' ) ;
#14436=ORIENTED_EDGE ( 'NONE', *, *, #10433, .T. ) ;
#14438=ORIENTED_EDGE ( 'NONE', *, *, #12669, .T. ) ;
#14439=FACE_BOUND ( 'NONE', #11488, .T. ) ;
#14443=CYLINDRICAL_SURFACE ( 'NONE', #2056, 2.649999999999985700 ) ;
#14444=DIRECTION ( 'NONE',  ( 1.000000000000000000, 0.000000000000000000, 0.000000000000000000 ) ) ;
#14445=ORIENTED_EDGE ( 'NONE', *, *, #6645, .F. ) ;
#14465=DIRECTION ( 'NONE',  ( -0.2873478855663453846, -0.9578262852211513190, -0.000000000000000000 ) ) ;
#14471=PRODUCT_DEFINITION_CONTEXT ( 'detailed design', #4340, 'design' ) ;
#14486=DIRECTION ( 'NONE',  ( -1.000000000000000000, -0.000000000000000000, -0.000000000000000000 ) ) ;
#14496=DIRECTION ( 'NONE',  ( 0.000000000000000000, 0.000000000000000000, 1.000000000000000000 ) ) ;
#14504=CARTESIAN_POINT ( 'NONE',  ( 139.8040310085880833, 355.9707293956415697, 190.0000000000000000 ) ) ;
#14510=VERTEX_POINT ( 'NONE', #1385 ) ;
#14522=SURFACE_STYLE_USAGE ( .BOTH. , #13195 ) ;
#14523=ORIENTED_EDGE ( 'NONE', *, *, #5928, .T. ) ;
#14524=VERTEX_POINT ( 'NONE', #10249 ) ;
#14528=CARTESIAN_POINT ( 'NONE',  ( 638.7884810776471340, 166.5485936625643717, -210.0000000000000000 ) ) ;
#14530=DIRECTION ( 'NONE',  ( -1.000000000000000000, 0.000000000000000000, 0.000000000000000000 ) ) ;
#14549=CARTESIAN_POINT ( 'NONE',  ( 590.0000000000000000, -9.999999999999944933, 190.0000000000000000 ) ) ;
#14550=EDGE_LOOP ( 'NONE', ( #14436, #11632 ) ) ;
#14559=VERTEX_POINT ( 'NONE', #1690 ) ;
#14569=CARTESIAN_POINT ( 'NONE',  ( 107.2182642636026202, 357.3942142120087055, 210.0000000000000000 ) ) ;
#14571=DIRECTION ( 'NONE',  ( 1.000000000000000000, 0.000000000000000000, 0.000000000000000000 ) ) ;
#14575=AXIS2_PLACEMENT_3D ( 'NONE', #9387, #210, #13749 ) ;
#14581=EDGE_LOOP ( 'NONE', ( #5832, #2084, #6635, #9974 ) ) ;
#14590=LINE ( 'NONE', #8014, #4298 ) ;
#14616=CARTESIAN_POINT ( 'NONE',  ( 459.7035746174795463, 294.6698471414878782, 190.0000000000000000 ) ) ;
#14647=COLOUR_RGB('Dark Blue',0.08,0.2,0.34);
#14648=FILL_AREA_STYLE_COLOUR('',#14647);
#14649=FILL_AREA_STYLE('',(#14648));
#14650=SURFACE_STYLE_FILL_AREA(#14649);
#14651=SURFACE_SIDE_STYLE('',(#14650));
#14652=SURFACE_STYLE_USAGE(.BOTH.,#14651);
#14653=PRESENTATION_STYLE_ASSIGNMENT((#14652));
ENDSEC;
END-ISO-10303-21;
